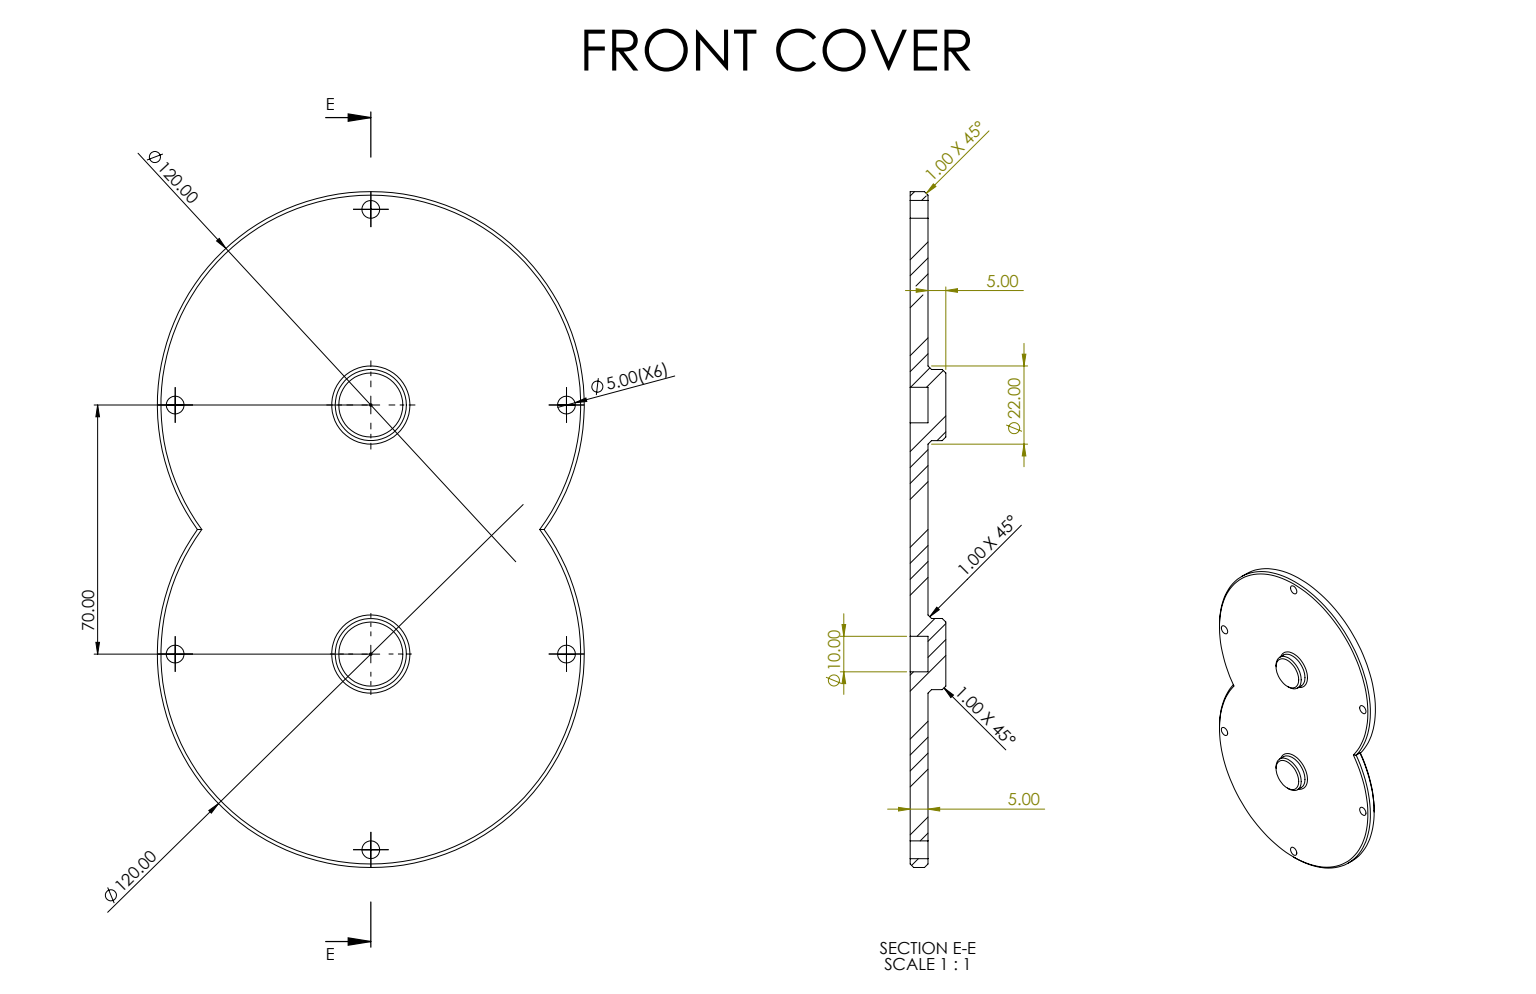
ISO-10303-21;
HEADER;
FILE_DESCRIPTION (('STEP AP214'),
    '1' );
FILE_NAME ('FRONT COVER.step',
    '2026-10-24T00:51:42',
    ( '' ),
    ( '' ),
    'SwSTEP 2.0',
    'SolidWorks 2025',
    '' );
FILE_SCHEMA (( 'AUTOMOTIVE_DESIGN' ));
ENDSEC;

DATA;
#13=ORIENTED_EDGE ( 'NONE', *, *, #8232, .T. ) ;
#20=CIRCLE ( 'NONE', #20518, 59.99999999999703704 ) ;
#28=DIRECTION ( 'NONE',  ( 0.000000000000000000, 1.000000000000000000, 0.000000000000000000 ) ) ;
#51=DIRECTION ( 'NONE',  ( 0.000000000000000000, 0.000000000000000000, -1.000000000000000000 ) ) ;
#74=VECTOR ( 'NONE', #6196, 1000.000000000000114 ) ;
#113=DIRECTION ( 'NONE',  ( 0.000000000000000000, 0.000000000000000000, 1.000000000000000000 ) ) ;
#181=DIRECTION ( 'NONE',  ( 8.659560562354903276E-17, -0.7071067811865500152, 0.7071067811865451302 ) ) ;
#196=EDGE_CURVE ( 'NONE', #9340, #20230, #6736, .T. ) ;
#205=CYLINDRICAL_SURFACE ( 'NONE', #8297, 59.99999999999700862 ) ;
#210=CARTESIAN_POINT ( 'NONE',  ( 35.00000000000001421, 5.000000000000000000, 1.540743955509788682E-30 ) ) ;
#215=DIRECTION ( 'NONE',  ( 0.000000000000000000, 1.000000000000000000, 0.000000000000000000 ) ) ;
#224=ORIENTED_EDGE ( 'NONE', *, *, #266, .F. ) ;
#225=CARTESIAN_POINT ( 'NONE',  ( 35.00000000000001421, 5.000000000000000000, 1.540743955509788682E-30 ) ) ;
#227=CARTESIAN_POINT ( 'NONE',  ( -34.99999999999999289, 0.000000000000000000, -3.012171160963566127E-14 ) ) ;
#265=CYLINDRICAL_SURFACE ( 'NONE', #18235, 10.00000000000000000 ) ;
#266=EDGE_CURVE ( 'NONE', #2332, #7531, #8895, .T. ) ;
#277=ADVANCED_FACE ( 'NONE', ( #12548, #8677, #5469, #19561, #10835, #1813, #15871, #8796, #9131 ), #15657, .T. ) ;
#288=DIRECTION ( 'NONE',  ( 0.000000000000000000, 0.000000000000000000, -1.000000000000000000 ) ) ;
#300=CARTESIAN_POINT ( 'NONE',  ( -34.99999999999999289, -5.000000000000000000, -54.99999999999705125 ) ) ;
#347=DIRECTION ( 'NONE',  ( 0.000000000000000000, 1.000000000000000000, 0.000000000000000000 ) ) ;
#353=VERTEX_POINT ( 'NONE', #21620 ) ;
#368=EDGE_LOOP ( 'NONE', ( #6095, #15311 ) ) ;
#460=ORIENTED_EDGE ( 'NONE', *, *, #7404, .T. ) ;
#474=CONICAL_SURFACE ( 'NONE', #18047, 58.99999999999701572, 0.7853981633974447263 ) ;
#508=ORIENTED_EDGE ( 'NONE', *, *, #14045, .T. ) ;
#516=CARTESIAN_POINT ( 'NONE',  ( -34.99999999999999289, 0.000000000000000000, -3.012171160963566127E-14 ) ) ;
#534=ORIENTED_EDGE ( 'NONE', *, *, #12604, .F. ) ;
#595=CIRCLE ( 'NONE', #3894, 10.00000000000000000 ) ;
#616=FACE_OUTER_BOUND ( 'NONE', #2436, .T. ) ;
#624=AXIS2_PLACEMENT_3D ( 'NONE', #14990, #8139, #11902 ) ;
#635=VECTOR ( 'NONE', #1063, 1000.000000000000114 ) ;
#664=DIRECTION ( 'NONE',  ( 0.000000000000000000, 1.000000000000000000, 0.000000000000000000 ) ) ;
#672=CARTESIAN_POINT ( 'NONE',  ( 34.99999999999999289, 0.000000000000000000, -57.49999999999705835 ) ) ;
#699=LINE ( 'NONE', #7682, #18205 ) ;
#717=ORIENTED_EDGE ( 'NONE', *, *, #8304, .F. ) ;
#734=ORIENTED_EDGE ( 'NONE', *, *, #2868, .F. ) ;
#762=DIRECTION ( 'NONE',  ( 0.000000000000000000, 1.000000000000000000, 0.000000000000000000 ) ) ;
#805=ADVANCED_FACE ( 'NONE', ( #10988 ), #3257, .T. ) ;
#830=ORIENTED_EDGE ( 'NONE', *, *, #3767, .F. ) ;
#840=CARTESIAN_POINT ( 'NONE',  ( -0.2854126906103648387, -4.332981472378772736, -48.52899265465751455 ) ) ;
#864=CARTESIAN_POINT ( 'NONE',  ( -89.99999999999701572, -5.000000000000000000, -3.012171160963566127E-14 ) ) ;
#904=EDGE_CURVE ( 'NONE', #353, #12856, #6012, .T. ) ;
#944=CARTESIAN_POINT ( 'NONE',  ( 34.99999999999999289, -5.000000000000000000, -54.99999999999705835 ) ) ;
#950=VERTEX_POINT ( 'NONE', #9985 ) ;
#959=ORIENTED_EDGE ( 'NONE', *, *, #1342, .F. ) ;
#960=UNCERTAINTY_MEASURE_WITH_UNIT (LENGTH_MEASURE( 1.000000000000000082E-05 ), #19624, 'distance_accuracy_value', 'NONE');
#982=EDGE_LOOP ( 'NONE', ( #22438, #1446 ) ) ;
#993=ORIENTED_EDGE ( 'NONE', *, *, #18740, .F. ) ;
#997=CARTESIAN_POINT ( 'NONE',  ( -34.99999999999999289, 0.000000000000000000, -58.99999999999701572 ) ) ;
#1011=CARTESIAN_POINT ( 'NONE',  ( 35.00000000000001421, -5.000000000000000000, 1.540743955509788682E-30 ) ) ;
#1015=ORIENTED_EDGE ( 'NONE', *, *, #2081, .T. ) ;
#1027=DIRECTION ( 'NONE',  ( 0.000000000000000000, -1.000000000000000000, 0.000000000000000000 ) ) ;
#1035=DIRECTION ( 'NONE',  ( 5.292376706370188309E-15, 0.000000000000000000, 1.000000000000000000 ) ) ;
#1039=FACE_OUTER_BOUND ( 'NONE', #8515, .T. ) ;
#1063=DIRECTION ( 'NONE',  ( 0.000000000000000000, 0.7071067811865549002, 0.7071067811865402453 ) ) ;
#1065=ORIENTED_EDGE ( 'NONE', *, *, #16608, .T. ) ;
#1105=AXIS2_PLACEMENT_3D ( 'NONE', #8719, #1616, #8487 ) ;
#1153=DIRECTION ( 'NONE',  ( 0.000000000000000000, 1.000000000000000000, 0.000000000000000000 ) ) ;
#1160=ADVANCED_FACE ( 'NONE', ( #14426 ), #18742, .T. ) ;
#1180=DIRECTION ( 'NONE',  ( 0.000000000000000000, 1.000000000000000000, 0.000000000000000000 ) ) ;
#1201=ADVANCED_FACE ( 'NONE', ( #7344 ), #11115, .F. ) ;
#1208=ORIENTED_EDGE ( 'NONE', *, *, #15769, .F. ) ;
#1214=VECTOR ( 'NONE', #15855, 1000.000000000000000 ) ;
#1223=CARTESIAN_POINT ( 'NONE',  ( -0.5687583343899673682, -4.666323447581315342, 48.32169744526331812 ) ) ;
#1247=CARTESIAN_POINT ( 'NONE',  ( 89.99999999999701572, 0.000000000000000000, -2.500000000000060840 ) ) ;
#1252=ORIENTED_EDGE ( 'NONE', *, *, #21699, .F. ) ;
#1259=ORIENTED_EDGE ( 'NONE', *, *, #15717, .F. ) ;
#1264=EDGE_CURVE ( 'NONE', #4080, #2931, #22007, .T. ) ;
#1272=LINE ( 'NONE', #4387, #9795 ) ;
#1273=CARTESIAN_POINT ( 'NONE',  ( -34.99999999999999289, -1.000000000000028644, -3.012171160963566127E-14 ) ) ;
#1277=VERTEX_POINT ( 'NONE', #9857 ) ;
#1313=VECTOR ( 'NONE', #19787, 1000.000000000000000 ) ;
#1321=LINE ( 'NONE', #11407, #12067 ) ;
#1333=EDGE_CURVE ( 'NONE', #7707, #18834, #16846, .T. ) ;
#1342=EDGE_CURVE ( 'NONE', #6332, #11390, #20202, .T. ) ;
#1345=ORIENTED_EDGE ( 'NONE', *, *, #1728, .F. ) ;
#1351=CARTESIAN_POINT ( 'NONE',  ( -34.99999999999999289, 0.000000000000000000, -54.99999999999705125 ) ) ;
#1357=ORIENTED_EDGE ( 'NONE', *, *, #7511, .T. ) ;
#1360=ORIENTED_EDGE ( 'NONE', *, *, #8232, .F. ) ;
#1361=DIRECTION ( 'NONE',  ( 0.000000000000000000, 0.000000000000000000, 1.000000000000000000 ) ) ;
#1377=EDGE_CURVE ( 'NONE', #9166, #8764, #11774, .T. ) ;
#1381=AXIS2_PLACEMENT_3D ( 'NONE', #8599, #1617, #10533 ) ;
#1419=ORIENTED_EDGE ( 'NONE', *, *, #5332, .F. ) ;
#1421=ORIENTED_EDGE ( 'NONE', *, *, #8605, .F. ) ;
#1422=EDGE_CURVE ( 'NONE', #6590, #6061, #10662, .T. ) ;
#1424=DIRECTION ( 'NONE',  ( 0.000000000000000000, 0.000000000000000000, -1.000000000000000000 ) ) ;
#1446=ORIENTED_EDGE ( 'NONE', *, *, #8571, .T. ) ;
#1452=B_SPLINE_CURVE_WITH_KNOTS ( 'NONE', 3,
 ( #13805, #20822, #11366, #2671 ),
 .UNSPECIFIED., .F., .F.,
 ( 4, 4 ),
 ( 0.000000000000000000, 0.001590342073036659634 ),
 .UNSPECIFIED. ) ;
#1490=FACE_OUTER_BOUND ( 'NONE', #12539, .T. ) ;
#1500=VERTEX_POINT ( 'NONE', #10137 ) ;
#1504=DIRECTION ( 'NONE',  ( 0.000000000000000000, 1.000000000000000000, 0.000000000000000000 ) ) ;
#1519=ORIENTED_EDGE ( 'NONE', *, *, #4640, .F. ) ;
#1543=CARTESIAN_POINT ( 'NONE',  ( 35.00000000000002132, -5.000000000000000000, -59.99999999999703704 ) ) ;
#1559=CARTESIAN_POINT ( 'NONE',  ( -34.99999999999999289, -5.000000000000000000, -52.49999999999705125 ) ) ;
#1604=DIRECTION ( 'NONE',  ( 0.000000000000000000, 0.000000000000000000, 1.000000000000000000 ) ) ;
#1616=DIRECTION ( 'NONE',  ( 0.000000000000000000, 1.000000000000000000, 0.000000000000000000 ) ) ;
#1617=DIRECTION ( 'NONE',  ( 0.000000000000000000, -1.000000000000000000, 0.000000000000000000 ) ) ;
#1637=DIRECTION ( 'NONE',  ( 0.000000000000000000, 1.000000000000000000, 0.000000000000000000 ) ) ;
#1648=CARTESIAN_POINT ( 'NONE',  ( 0.000000000000000000, 0.000000000000000000, 0.000000000000000000 ) ) ;
#1660=DIRECTION ( 'NONE',  ( 0.000000000000000000, 0.000000000000000000, -1.000000000000000000 ) ) ;
#1671=ORIENTED_EDGE ( 'NONE', *, *, #14527, .T. ) ;
#1675=AXIS2_PLACEMENT_3D ( 'NONE', #11723, #4855, #15373 ) ;
#1685=ORIENTED_EDGE ( 'NONE', *, *, #19206, .T. ) ;
#1689=DIRECTION ( 'NONE',  ( 0.000000000000000000, 1.000000000000000000, 0.000000000000000000 ) ) ;
#1710=LINE ( 'NONE', #16802, #7044 ) ;
#1711=LINE ( 'NONE', #14047, #14166 ) ;
#1717=DIRECTION ( 'NONE',  ( 0.000000000000000000, 1.000000000000000000, 0.000000000000000000 ) ) ;
#1728=EDGE_CURVE ( 'NONE', #11390, #6332, #7045, .T. ) ;
#1733=FACE_OUTER_BOUND ( 'NONE', #6732, .T. ) ;
#1757=AXIS2_PLACEMENT_3D ( 'NONE', #9404, #14192, #10999 ) ;
#1767=VERTEX_POINT ( 'NONE', #11621 ) ;
#1778=VECTOR ( 'NONE', #2503, 1000.000000000000000 ) ;
#1791=AXIS2_PLACEMENT_3D ( 'NONE', #4033, #12375, #113 ) ;
#1813=FACE_BOUND ( 'NONE', #15683, .T. ) ;
#1839=EDGE_CURVE ( 'NONE', #3030, #17217, #20670, .T. ) ;
#1853=CARTESIAN_POINT ( 'NONE',  ( -34.99999999999999289, -5.000000000000000000, 4.999999999999969802 ) ) ;
#1867=AXIS2_PLACEMENT_3D ( 'NONE', #14446, #11021, #16064 ) ;
#1901=LINE ( 'NONE', #8880, #1214 ) ;
#1902=ADVANCED_FACE ( 'NONE', ( #11839 ), #12486, .T. ) ;
#1946=DIRECTION ( 'NONE',  ( 0.000000000000000000, 0.000000000000000000, 1.000000000000000000 ) ) ;
#1951=FACE_BOUND ( 'NONE', #22385, .T. ) ;
#1952=AXIS2_PLACEMENT_3D ( 'NONE', #9959, #4929, #22467 ) ;
#1967=AXIS2_PLACEMENT_3D ( 'NONE', #22562, #6856, #13822 ) ;
#1970=CIRCLE ( 'NONE', #3085, 4.999999999999997335 ) ;
#1987=EDGE_CURVE ( 'NONE', #9166, #6590, #21289, .T. ) ;
#2033=CARTESIAN_POINT ( 'NONE',  ( 34.99999999999999289, 0.000000000000000000, -54.99999999999705835 ) ) ;
#2036=CARTESIAN_POINT ( 'NONE',  ( 35.00000000000001421, 5.000000000000000000, 1.540743955509788682E-30 ) ) ;
#2064=DIRECTION ( 'NONE',  ( 0.000000000000000000, 1.000000000000000000, 0.000000000000000000 ) ) ;
#2074=ORIENTED_EDGE ( 'NONE', *, *, #1422, .T. ) ;
#2080=LINE ( 'NONE', #5746, #14555 ) ;
#2081=EDGE_CURVE ( 'NONE', #10039, #14190, #11408, .T. ) ;
#2085=ORIENTED_EDGE ( 'NONE', *, *, #12937, .F. ) ;
#2100=CARTESIAN_POINT ( 'NONE',  ( 35.00000000000001421, -5.000000000000000000, 4.999999999999997335 ) ) ;
#2102=ORIENTED_EDGE ( 'NONE', *, *, #14902, .T. ) ;
#2105=LINE ( 'NONE', #14117, #16305 ) ;
#2113=AXIS2_PLACEMENT_3D ( 'NONE', #6299, #2756, #13257 ) ;
#2123=ORIENTED_EDGE ( 'NONE', *, *, #4379, .T. ) ;
#2142=DIRECTION ( 'NONE',  ( 0.000000000000000000, 1.000000000000000000, 0.000000000000000000 ) ) ;
#2199=VERTEX_POINT ( 'NONE', #15694 ) ;
#2204=( NAMED_UNIT ( * ) PLANE_ANGLE_UNIT ( ) SI_UNIT ( $, .RADIAN. ) );
#2205=ORIENTED_EDGE ( 'NONE', *, *, #15691, .F. ) ;
#2234=ORIENTED_EDGE ( 'NONE', *, *, #20437, .T. ) ;
#2261=DIRECTION ( 'NONE',  ( 0.000000000000000000, 1.000000000000000000, 0.000000000000000000 ) ) ;
#2285=ORIENTED_EDGE ( 'NONE', *, *, #3044, .T. ) ;
#2310=EDGE_LOOP ( 'NONE', ( #20692, #6820, #17268, #1015, #21602, #6129 ) ) ;
#2332=VERTEX_POINT ( 'NONE', #12582 ) ;
#2341=ADVANCED_FACE ( 'NONE', ( #16259 ), #19718, .T. ) ;
#2357=DIRECTION ( 'NONE',  ( 0.000000000000000000, 0.000000000000000000, 1.000000000000000000 ) ) ;
#2392=CARTESIAN_POINT ( 'NONE',  ( -34.99999999999999289, -3.999999999999985345, -3.012171160963566127E-14 ) ) ;
#2393=CONICAL_SURFACE ( 'NONE', #10411, 59.99999999999700862, 0.7853981633974380649 ) ;
#2396=AXIS2_PLACEMENT_3D ( 'NONE', #17885, #21211, #7342 ) ;
#2419=AXIS2_PLACEMENT_3D ( 'NONE', #20940, #1689, #8221 ) ;
#2427=EDGE_CURVE ( 'NONE', #22344, #3030, #8546, .T. ) ;
#2436=EDGE_LOOP ( 'NONE', ( #20453, #6374, #6252, #19334 ) ) ;
#2458=CARTESIAN_POINT ( 'NONE',  ( -34.99999999999999289, 0.000000000000000000, -3.012171160963566127E-14 ) ) ;
#2460=ORIENTED_EDGE ( 'NONE', *, *, #10047, .T. ) ;
#2472=VERTEX_POINT ( 'NONE', #1559 ) ;
#2484=CYLINDRICAL_SURFACE ( 'NONE', #16671, 59.99999999999703704 ) ;
#2503=DIRECTION ( 'NONE',  ( -0.000000000000000000, -1.000000000000000000, -0.000000000000000000 ) ) ;
#2523=ORIENTED_EDGE ( 'NONE', *, *, #16926, .T. ) ;
#2529=DIRECTION ( 'NONE',  ( 0.000000000000000000, 0.000000000000000000, 1.000000000000000000 ) ) ;
#2548=PRODUCT ( 'FRONT COVER', 'FRONT COVER', '', ( #6769 ) ) ;
#2564=CARTESIAN_POINT ( 'NONE',  ( -34.99999999999999289, 0.000000000000000000, -57.49999999999705125 ) ) ;
#2596=EDGE_CURVE ( 'NONE', #14190, #8015, #20812, .T. ) ;
#2643=PLANE ( 'NONE',  #3678 ) ;
#2671=CARTESIAN_POINT ( 'NONE',  ( -2.783226368218592341E-14, 0.000000000000000000, 47.49736834814792985 ) ) ;
#2688=DIRECTION ( 'NONE',  ( 0.000000000000000000, 0.000000000000000000, 1.000000000000000000 ) ) ;
#2706=CIRCLE ( 'NONE', #22101, 11.00000000000003730 ) ;
#2710=DIRECTION ( 'NONE',  ( 0.000000000000000000, 1.000000000000000000, 0.000000000000000000 ) ) ;
#2726=LINE ( 'NONE', #17958, #7374 ) ;
#2746=AXIS2_PLACEMENT_3D ( 'NONE', #6857, #22684, #20946 ) ;
#2756=DIRECTION ( 'NONE',  ( -0.000000000000000000, -1.000000000000000000, -0.000000000000000000 ) ) ;
#2782=ORIENTED_EDGE ( 'NONE', *, *, #14527, .F. ) ;
#2783=FACE_OUTER_BOUND ( 'NONE', #16329, .T. ) ;
#2790=EDGE_LOOP ( 'NONE', ( #508, #9529 ) ) ;
#2830=ORIENTED_EDGE ( 'NONE', *, *, #10117, .T. ) ;
#2836=DIRECTION ( 'NONE',  ( -0.000000000000000000, 1.000000000000000000, -0.000000000000000000 ) ) ;
#2840=VERTEX_POINT ( 'NONE', #20675 ) ;
#2863=VECTOR ( 'NONE', #17832, 1000.000000000000114 ) ;
#2867=DIRECTION ( 'NONE',  ( 1.734723475976892686E-15, 0.000000000000000000, 1.000000000000000000 ) ) ;
#2868=EDGE_CURVE ( 'NONE', #12296, #7531, #10896, .T. ) ;
#2875=VERTEX_POINT ( 'NONE', #15498 ) ;
#2891=EDGE_LOOP ( 'NONE', ( #17547, #17921, #11604, #5644 ) ) ;
#2908=DIRECTION ( 'NONE',  ( 0.000000000000000000, 1.000000000000000000, 0.000000000000000000 ) ) ;
#2909=DIRECTION ( 'NONE',  ( 0.000000000000000000, 1.000000000000000000, 0.000000000000000000 ) ) ;
#2931=VERTEX_POINT ( 'NONE', #4163 ) ;
#2972=ORIENTED_EDGE ( 'NONE', *, *, #3652, .F. ) ;
#2990=CARTESIAN_POINT ( 'NONE',  ( -34.99999999999998579, -3.999999999999985345, -59.99999999999703704 ) ) ;
#2996=EDGE_LOOP ( 'NONE', ( #4896, #14681, #2460, #14741, #12315, #14007 ) ) ;
#3001=ORIENTED_EDGE ( 'NONE', *, *, #3202, .F. ) ;
#3009=DIRECTION ( 'NONE',  ( -0.000000000000000000, 1.000000000000000000, -0.000000000000000000 ) ) ;
#3014=CARTESIAN_POINT ( 'NONE',  ( -34.99999999999999289, 4.000000000000028422, -3.012171160963566127E-14 ) ) ;
#3030=VERTEX_POINT ( 'NONE', #12739 ) ;
#3044=EDGE_CURVE ( 'NONE', #4376, #13677, #16435, .T. ) ;
#3050=EDGE_LOOP ( 'NONE', ( #11360, #15711 ) ) ;
#3077=VERTEX_POINT ( 'NONE', #9876 ) ;
#3085=AXIS2_PLACEMENT_3D ( 'NONE', #4024, #9509, #21544 ) ;
#3097=ORIENTED_EDGE ( 'NONE', *, *, #1333, .F. ) ;
#3111=FACE_OUTER_BOUND ( 'NONE', #22167, .T. ) ;
#3131=DIRECTION ( 'NONE',  ( 0.000000000000000000, 0.000000000000000000, 1.000000000000000000 ) ) ;
#3142=ORIENTED_EDGE ( 'NONE', *, *, #8081, .T. ) ;
#3143=B_SPLINE_CURVE_WITH_KNOTS ( 'NONE', 3,
 ( #16538, #20211, #840, #21819 ),
 .UNSPECIFIED., .F., .F.,
 ( 4, 4 ),
 ( 0.000000000000000000, 0.001452302087772874839 ),
 .UNSPECIFIED. ) ;
#3148=EDGE_LOOP ( 'NONE', ( #12892, #6241 ) ) ;
#3164=ADVANCED_FACE ( 'NONE', ( #2783 ), #9475, .T. ) ;
#3187=ORIENTED_EDGE ( 'NONE', *, *, #12577, .F. ) ;
#3202=EDGE_CURVE ( 'NONE', #4584, #7707, #16799, .T. ) ;
#3206=AXIS2_PLACEMENT_3D ( 'NONE', #16063, #3935, #17905 ) ;
#3215=CIRCLE ( 'NONE', #2113, 11.00000000000003730 ) ;
#3219=EDGE_LOOP ( 'NONE', ( #15771, #11245, #13002, #1519 ) ) ;
#3244=EDGE_LOOP ( 'NONE', ( #15424, #19591 ) ) ;
#3257=CYLINDRICAL_SURFACE ( 'NONE', #3822, 10.00000000000000000 ) ;
#3280=CARTESIAN_POINT ( 'NONE',  ( 89.99999999999701572, 0.000000000000000000, -5.216535399428728743E-14 ) ) ;
#3331=CARTESIAN_POINT ( 'NONE',  ( -34.99999999999999289, -5.000000000000000000, -3.012171160963566127E-14 ) ) ;
#3332=ORIENTED_EDGE ( 'NONE', *, *, #6770, .F. ) ;
#3370=EDGE_LOOP ( 'NONE', ( #18621, #9458 ) ) ;
#3408=DIRECTION ( 'NONE',  ( 0.000000000000000000, 0.000000000000000000, 1.000000000000000000 ) ) ;
#3410=DIRECTION ( 'NONE',  ( 0.000000000000000000, 1.000000000000000000, 0.000000000000000000 ) ) ;
#3419=ADVANCED_FACE ( 'NONE', ( #10639, #10997, #21097, #21428, #1951, #12818, #7563, #10877, #5396 ), #19830, .F. ) ;
#3431=DIRECTION ( 'NONE',  ( 0.000000000000000000, 1.000000000000000000, 0.000000000000000000 ) ) ;
#3436=EDGE_CURVE ( 'NONE', #2840, #5633, #16413, .T. ) ;
#3441=AXIS2_PLACEMENT_3D ( 'NONE', #210, #7322, #9038 ) ;
#3444=VECTOR ( 'NONE', #1153, 1000.000000000000000 ) ;
#3454=SHAPE_DEFINITION_REPRESENTATION ( #16821, #13507 ) ;
#3460=DIRECTION ( 'NONE',  ( 0.000000000000000000, -1.000000000000000000, 0.000000000000000000 ) ) ;
#3496=VERTEX_POINT ( 'NONE', #14304 ) ;
#3524=ORIENTED_EDGE ( 'NONE', *, *, #4411, .F. ) ;
#3525=DIRECTION ( 'NONE',  ( 0.000000000000000000, 1.000000000000000000, -0.000000000000000000 ) ) ;
#3528=B_SPLINE_CURVE_WITH_KNOTS ( 'NONE', 3,
 ( #6847, #8220, #1223, #11762 ),
 .UNSPECIFIED., .F., .F.,
 ( 4, 4 ),
 ( 0.000000000000000000, 0.001452302087772880043 ),
 .UNSPECIFIED. ) ;
#3530=DIRECTION ( 'NONE',  ( 0.000000000000000000, 0.000000000000000000, 1.000000000000000000 ) ) ;
#3563=DIRECTION ( 'NONE',  ( 0.000000000000000000, 1.000000000000000000, 0.000000000000000000 ) ) ;
#3570=DIRECTION ( 'NONE',  ( 0.000000000000000000, 1.000000000000000000, 0.000000000000000000 ) ) ;
#3581=DIRECTION ( 'NONE',  ( 0.000000000000000000, 1.000000000000000000, 0.000000000000000000 ) ) ;
#3631=AXIS2_PLACEMENT_3D ( 'NONE', #16764, #9658, #8064 ) ;
#3652=EDGE_CURVE ( 'NONE', #11550, #1500, #6318, .T. ) ;
#3659=ORIENTED_EDGE ( 'NONE', *, *, #266, .T. ) ;
#3664=FACE_OUTER_BOUND ( 'NONE', #2790, .T. ) ;
#3678=AXIS2_PLACEMENT_3D ( 'NONE', #19935, #8024, #14982 ) ;
#3711=DIRECTION ( 'NONE',  ( 0.000000000000000000, 0.000000000000000000, 1.000000000000000000 ) ) ;
#3730=CARTESIAN_POINT ( 'NONE',  ( -34.99999999999999289, -3.999999999999985345, -3.012171160963566127E-14 ) ) ;
#3742=CARTESIAN_POINT ( 'NONE',  ( -34.99999999999997868, 0.000000000000000000, 54.99999999999698730 ) ) ;
#3758=EDGE_LOOP ( 'NONE', ( #16747, #22171, #10337, #18642 ) ) ;
#3767=EDGE_CURVE ( 'NONE', #21906, #4376, #1710, .T. ) ;
#3790=DIRECTION ( 'NONE',  ( 0.000000000000000000, 0.000000000000000000, 1.000000000000000000 ) ) ;
#3813=ORIENTED_EDGE ( 'NONE', *, *, #19503, .T. ) ;
#3815=EDGE_LOOP ( 'NONE', ( #2074, #13522, #4848, #12384 ) ) ;
#3822=AXIS2_PLACEMENT_3D ( 'NONE', #16250, #17976, #6919 ) ;
#3849=DIRECTION ( 'NONE',  ( 0.000000000000000000, 0.000000000000000000, 1.000000000000000000 ) ) ;
#3894=AXIS2_PLACEMENT_3D ( 'NONE', #11883, #13478, #13700 ) ;
#3907=CARTESIAN_POINT ( 'NONE',  ( -34.99999999999999289, -5.000000000000000000, -3.012171160963566127E-14 ) ) ;
#3913=FACE_OUTER_BOUND ( 'NONE', #19433, .T. ) ;
#3916=DIRECTION ( 'NONE',  ( 0.000000000000000000, -1.000000000000000000, 0.000000000000000000 ) ) ;
#3922=ORIENTED_EDGE ( 'NONE', *, *, #4411, .T. ) ;
#3930=VERTEX_POINT ( 'NONE', #19360 ) ;
#3932=EDGE_CURVE ( 'NONE', #20230, #4376, #10098, .T. ) ;
#3935=DIRECTION ( 'NONE',  ( 0.000000000000000000, 1.000000000000000000, 0.000000000000000000 ) ) ;
#3944=ADVANCED_FACE ( 'NONE', ( #3664 ), #10615, .F. ) ;
#3963=AXIS2_PLACEMENT_3D ( 'NONE', #9358, #2142, #12886 ) ;
#3976=AXIS2_PLACEMENT_3D ( 'NONE', #8325, #2836, #6606 ) ;
#3982=AXIS2_PLACEMENT_3D ( 'NONE', #19031, #18371, #2688 ) ;
#3993=ORIENTED_EDGE ( 'NONE', *, *, #17293, .T. ) ;
#3996=AXIS2_PLACEMENT_3D ( 'NONE', #4739, #4618, #18250 ) ;
#4011=DIRECTION ( 'NONE',  ( -0.000000000000000000, 1.000000000000000000, -0.000000000000000000 ) ) ;
#4024=CARTESIAN_POINT ( 'NONE',  ( 35.00000000000001421, -5.000000000000000000, 1.540743955509788682E-30 ) ) ;
#4033=CARTESIAN_POINT ( 'NONE',  ( -34.99999999999999289, 4.000000000000028422, -3.012171160963566127E-14 ) ) ;
#4057=DIRECTION ( 'NONE',  ( 0.000000000000000000, 0.000000000000000000, 1.000000000000000000 ) ) ;
#4061=EDGE_LOOP ( 'NONE', ( #18011, #5121, #2523, #959 ) ) ;
#4063=CARTESIAN_POINT ( 'NONE',  ( -89.99999999999701572, 0.000000000000000000, 2.499999999999978684 ) ) ;
#4080=VERTEX_POINT ( 'NONE', #10264 ) ;
#4085=DIRECTION ( 'NONE',  ( 0.000000000000000000, 1.000000000000000000, 0.000000000000000000 ) ) ;
#4089=DIRECTION ( 'NONE',  ( -0.000000000000000000, -1.000000000000000000, -0.000000000000000000 ) ) ;
#4102=FACE_OUTER_BOUND ( 'NONE', #4209, .T. ) ;
#4132=DIRECTION ( 'NONE',  ( 0.000000000000000000, -0.000000000000000000, 1.000000000000000000 ) ) ;
#4137=CARTESIAN_POINT ( 'NONE',  ( -34.99999999999999289, 0.000000000000000000, -3.012171160963566127E-14 ) ) ;
#4153=ORIENTED_EDGE ( 'NONE', *, *, #15425, .T. ) ;
#4163=CARTESIAN_POINT ( 'NONE',  ( -34.99999999999999289, 0.000000000000000000, -11.00000000000006750 ) ) ;
#4201=CARTESIAN_POINT ( 'NONE',  ( 35.00000000000001421, -5.000000000000000000, 1.540743955509788682E-30 ) ) ;
#4209=EDGE_LOOP ( 'NONE', ( #11237, #6980, #15911, #7527 ) ) ;
#4211=CARTESIAN_POINT ( 'NONE',  ( 35.00000000000002132, -5.000000000000000000, -59.99999999999703704 ) ) ;
#4218=DIRECTION ( 'NONE',  ( 0.000000000000000000, 0.000000000000000000, 1.000000000000000000 ) ) ;
#4225=CARTESIAN_POINT ( 'NONE',  ( -34.99999999999999289, -5.000000000000000000, -54.99999999999705125 ) ) ;
#4235=AXIS2_PLACEMENT_3D ( 'NONE', #7172, #21047, #9126 ) ;
#4243=VECTOR ( 'NONE', #17120, 1000.000000000000000 ) ;
#4244=FACE_OUTER_BOUND ( 'NONE', #3050, .T. ) ;
#4250=DIRECTION ( 'NONE',  ( -0.000000000000000000, -1.000000000000000000, -0.000000000000000000 ) ) ;
#4254=CARTESIAN_POINT ( 'NONE',  ( 35.00000000000001421, 0.000000000000000000, 1.540743955509788682E-30 ) ) ;
#4257=DIRECTION ( 'NONE',  ( 0.000000000000000000, 0.000000000000000000, -1.000000000000000000 ) ) ;
#4311=ORIENTED_EDGE ( 'NONE', *, *, #5518, .F. ) ;
#4316=AXIS2_PLACEMENT_3D ( 'NONE', #18352, #3009, #13069 ) ;
#4322=CIRCLE ( 'NONE', #22253, 2.500000000000002220 ) ;
#4333=LINE ( 'NONE', #997, #6879 ) ;
#4341=DIRECTION ( 'NONE',  ( 0.000000000000000000, 0.000000000000000000, 1.000000000000000000 ) ) ;
#4344=VERTEX_POINT ( 'NONE', #12840 ) ;
#4358=AXIS2_PLACEMENT_3D ( 'NONE', #18098, #347, #4132 ) ;
#4365=CARTESIAN_POINT ( 'NONE',  ( 35.00000000000001421, -1.000000000000028644, 1.540743955509788682E-30 ) ) ;
#4376=VERTEX_POINT ( 'NONE', #19627 ) ;
#4379=EDGE_CURVE ( 'NONE', #13224, #13528, #22248, .T. ) ;
#4383=AXIS2_PLACEMENT_3D ( 'NONE', #15739, #12089, #51 ) ;
#4387=CARTESIAN_POINT ( 'NONE',  ( -34.99999999999998579, -3.999999999999985345, -59.99999999999703704 ) ) ;
#4411=EDGE_CURVE ( 'NONE', #13828, #11150, #1272, .T. ) ;
#4429=DIRECTION ( 'NONE',  ( 0.000000000000000000, 0.000000000000000000, 1.000000000000000000 ) ) ;
#4444=AXIS2_PLACEMENT_3D ( 'NONE', #1273, #6553, #13957 ) ;
#4445=DIRECTION ( 'NONE',  ( 0.000000000000000000, 0.000000000000000000, 1.000000000000000000 ) ) ;
#4458=CYLINDRICAL_SURFACE ( 'NONE', #14761, 59.99999999999703704 ) ;
#4539=AXIS2_PLACEMENT_3D ( 'NONE', #8996, #21607, #288 ) ;
#4543=DIRECTION ( 'NONE',  ( 0.000000000000000000, 1.000000000000000000, 0.000000000000000000 ) ) ;
#4558=DIRECTION ( 'NONE',  ( 0.000000000000000000, 0.000000000000000000, 1.000000000000000000 ) ) ;
#4584=VERTEX_POINT ( 'NONE', #17075 ) ;
#4606=AXIS2_PLACEMENT_3D ( 'NONE', #17348, #8424, #15393 ) ;
#4618=DIRECTION ( 'NONE',  ( 0.000000000000000000, -1.000000000000000000, 0.000000000000000000 ) ) ;
#4619=CARTESIAN_POINT ( 'NONE',  ( 35.00000000000001421, 5.000000000000000000, 9.000000000000035527 ) ) ;
#4640=EDGE_CURVE ( 'NONE', #15853, #12856, #2726, .T. ) ;
#4681=CYLINDRICAL_SURFACE ( 'NONE', #11906, 4.999999999999997335 ) ;
#4682=ADVANCED_FACE ( 'NONE', ( #6273 ), #16811, .T. ) ;
#4689=DIRECTION ( 'NONE',  ( 0.000000000000000000, 1.000000000000000000, 0.000000000000000000 ) ) ;
#4715=CARTESIAN_POINT ( 'NONE',  ( -34.99999999999999289, 0.000000000000000000, -52.49999999999705125 ) ) ;
#4729=ORIENTED_EDGE ( 'NONE', *, *, #3652, .T. ) ;
#4739=CARTESIAN_POINT ( 'NONE',  ( -34.99999999999999289, 5.000000000000000000, -3.012171160963566127E-14 ) ) ;
#4781=CIRCLE ( 'NONE', #7695, 5.000000000000000000 ) ;
#4786=DIRECTION ( 'NONE',  ( 0.000000000000000000, 1.000000000000000000, 0.000000000000000000 ) ) ;
#4789=DIRECTION ( 'NONE',  ( 0.000000000000000000, 1.000000000000000000, 0.000000000000000000 ) ) ;
#4809=CARTESIAN_POINT ( 'NONE',  ( -34.99999999999999289, 0.000000000000000000, -3.012171160963566127E-14 ) ) ;
#4829=EDGE_CURVE ( 'NONE', #11055, #19583, #22454, .T. ) ;
#4834=CYLINDRICAL_SURFACE ( 'NONE', #1105, 2.500000000000002220 ) ;
#4848=ORIENTED_EDGE ( 'NONE', *, *, #8479, .T. ) ;
#4855=DIRECTION ( 'NONE',  ( -0.000000000000000000, -1.000000000000000000, -0.000000000000000000 ) ) ;
#4876=CARTESIAN_POINT ( 'NONE',  ( -34.99999999999999289, -5.000000000000000000, 59.99999999999698019 ) ) ;
#4887=ORIENTED_EDGE ( 'NONE', *, *, #11836, .F. ) ;
#4896=ORIENTED_EDGE ( 'NONE', *, *, #1987, .F. ) ;
#4929=DIRECTION ( 'NONE',  ( 0.000000000000000000, -1.000000000000000000, 0.000000000000000000 ) ) ;
#4935=CIRCLE ( 'NONE', #2746, 2.500000000000002220 ) ;
#4949=DIRECTION ( 'NONE',  ( 0.000000000000000000, 1.000000000000000000, 0.000000000000000000 ) ) ;
#4972=VERTEX_POINT ( 'NONE', #7972 ) ;
#4981=CARTESIAN_POINT ( 'NONE',  ( 89.99999999999701572, 0.000000000000000000, 2.499999999999956479 ) ) ;
#4987=ADVANCED_BREP_SHAPE_REPRESENTATION ( '', ( #10654, #18273 ), #22681 ) ;
#5004=VERTEX_POINT ( 'NONE', #4981 ) ;
#5020=EDGE_LOOP ( 'NONE', ( #15013, #11391 ) ) ;
#5038=CIRCLE ( 'NONE', #14531, 10.00000000000000000 ) ;
#5056=CARTESIAN_POINT ( 'NONE',  ( -34.99999999999999289, 5.000000000000000000, 9.000000000000007105 ) ) ;
#5105=ORIENTED_EDGE ( 'NONE', *, *, #10161, .T. ) ;
#5108=ORIENTED_EDGE ( 'NONE', *, *, #1839, .F. ) ;
#5110=FACE_OUTER_BOUND ( 'NONE', #2891, .T. ) ;
#5121=ORIENTED_EDGE ( 'NONE', *, *, #6388, .F. ) ;
#5140=CIRCLE ( 'NONE', #19411, 2.500000000000002220 ) ;
#5156=FACE_OUTER_BOUND ( 'NONE', #9966, .T. ) ;
#5169=CARTESIAN_POINT ( 'NONE',  ( 7.943521403985130338E-15, 0.000000000000000000, -47.49736834814795827 ) ) ;
#5178=CARTESIAN_POINT ( 'NONE',  ( 89.99999999999701572, 0.000000000000000000, -5.216535399428728743E-14 ) ) ;
#5244=CARTESIAN_POINT ( 'NONE',  ( 1.387778780781445676E-14, -5.000000000000000000, -48.73397172404115452 ) ) ;
#5246=DIRECTION ( 'NONE',  ( 0.000000000000000000, -1.000000000000000000, 0.000000000000000000 ) ) ;
#5275=EDGE_CURVE ( 'NONE', #11150, #10311, #18947, .T. ) ;
#5299=DIRECTION ( 'NONE',  ( 0.000000000000000000, 1.000000000000000000, 0.000000000000000000 ) ) ;
#5305=CARTESIAN_POINT ( 'NONE',  ( -34.99999999999999289, -3.999999999999985345, -3.012171160963566127E-14 ) ) ;
#5309=ORIENTED_EDGE ( 'NONE', *, *, #12414, .F. ) ;
#5332=EDGE_CURVE ( 'NONE', #8764, #10311, #11483, .T. ) ;
#5361=EDGE_CURVE ( 'NONE', #19717, #22344, #7818, .T. ) ;
#5388=DIRECTION ( 'NONE',  ( 0.000000000000000000, 0.000000000000000000, -1.000000000000000000 ) ) ;
#5391=FACE_OUTER_BOUND ( 'NONE', #16847, .T. ) ;
#5393=CARTESIAN_POINT ( 'NONE',  ( 35.00000000000001421, -5.000000000000000000, 1.540743955509788682E-30 ) ) ;
#5394=CONICAL_SURFACE ( 'NONE', #20045, 10.00000000000000000, 0.7853981633974447263 ) ;
#5396=FACE_OUTER_BOUND ( 'NONE', #2996, .T. ) ;
#5400=LINE ( 'NONE', #1853, #10060 ) ;
#5437=AXIS2_PLACEMENT_3D ( 'NONE', #11057, #4089, #16675 ) ;
#5469=FACE_BOUND ( 'NONE', #17372, .T. ) ;
#5474=CIRCLE ( 'NONE', #16448, 2.500000000000002220 ) ;
#5518=EDGE_CURVE ( 'NONE', #4344, #353, #17541, .T. ) ;
#5523=ORIENTED_EDGE ( 'NONE', *, *, #11051, .F. ) ;
#5532=DIRECTION ( 'NONE',  ( 0.000000000000000000, 1.000000000000000000, 0.000000000000000000 ) ) ;
#5547=EDGE_CURVE ( 'NONE', #4344, #15853, #13821, .T. ) ;
#5549=AXIS2_PLACEMENT_3D ( 'NONE', #21339, #16287, #14216 ) ;
#5574=VERTEX_POINT ( 'NONE', #1247 ) ;
#5590=DIRECTION ( 'NONE',  ( 0.000000000000000000, 0.000000000000000000, 1.000000000000000000 ) ) ;
#5633=VERTEX_POINT ( 'NONE', #9853 ) ;
#5644=ORIENTED_EDGE ( 'NONE', *, *, #5957, .F. ) ;
#5700=DIRECTION ( 'NONE',  ( 0.000000000000000000, 1.000000000000000000, -0.000000000000000000 ) ) ;
#5701=CYLINDRICAL_SURFACE ( 'NONE', #12448, 10.00000000000000000 ) ;
#5702=CARTESIAN_POINT ( 'NONE',  ( 35.00000000000001421, -1.000000000000028644, 1.540743955509788682E-30 ) ) ;
#5746=CARTESIAN_POINT ( 'NONE',  ( 35.00000000000001421, 5.000000000000000000, -10.00000000000000000 ) ) ;
#5804=AXIS2_PLACEMENT_3D ( 'NONE', #8668, #3525, #12106 ) ;
#5832=EDGE_CURVE ( 'NONE', #1767, #13224, #1711, .T. ) ;
#5839=CARTESIAN_POINT ( 'NONE',  ( -34.99999999999999289, 0.000000000000000000, -3.012171160963566127E-14 ) ) ;
#5890=CARTESIAN_POINT ( 'NONE',  ( 35.00000000000000000, -5.000000000000000000, 54.99999999999698019 ) ) ;
#5911=ORIENTED_EDGE ( 'NONE', *, *, #16926, .F. ) ;
#5913=LINE ( 'NONE', #12879, #7242 ) ;
#5915=DIRECTION ( 'NONE',  ( 0.000000000000000000, 1.000000000000000000, 0.000000000000000000 ) ) ;
#5926=CARTESIAN_POINT ( 'NONE',  ( -3.469446951953614189E-14, -3.999999999999985345, 48.73397172404114031 ) ) ;
#5932=CARTESIAN_POINT ( 'NONE',  ( -34.99999999999999289, -3.999999999999985345, -3.012171160963566127E-14 ) ) ;
#5957=EDGE_CURVE ( 'NONE', #2840, #4080, #14512, .T. ) ;
#6012=CIRCLE ( 'NONE', #15868, 2.500000000000002220 ) ;
#6022=CARTESIAN_POINT ( 'NONE',  ( -34.99999999999999289, 5.000000000000000000, -3.012171160963566127E-14 ) ) ;
#6061=VERTEX_POINT ( 'NONE', #1543 ) ;
#6089=CIRCLE ( 'NONE', #13752, 2.500000000000002220 ) ;
#6095=ORIENTED_EDGE ( 'NONE', *, *, #11836, .T. ) ;
#6100=CYLINDRICAL_SURFACE ( 'NONE', #11363, 2.500000000000002220 ) ;
#6119=CIRCLE ( 'NONE', #17763, 59.99999999999700862 ) ;
#6129=ORIENTED_EDGE ( 'NONE', *, *, #15717, .T. ) ;
#6141=ORIENTED_EDGE ( 'NONE', *, *, #1987, .T. ) ;
#6149=CARTESIAN_POINT ( 'NONE',  ( -34.99999999999999289, 1.000000000000044187, 9.999999999999971578 ) ) ;
#6162=DIRECTION ( 'NONE',  ( 0.000000000000000000, 1.000000000000000000, 0.000000000000000000 ) ) ;
#6169=FACE_OUTER_BOUND ( 'NONE', #4061, .T. ) ;
#6175=FACE_OUTER_BOUND ( 'NONE', #22032, .T. ) ;
#6179=CARTESIAN_POINT ( 'NONE',  ( -34.99999999999999289, 0.000000000000000000, -58.99999999999702993 ) ) ;
#6184=ADVANCED_FACE ( 'NONE', ( #5110 ), #265, .T. ) ;
#6196=DIRECTION ( 'NONE',  ( 0.000000000000000000, -0.7071067811865500152, -0.7071067811865451302 ) ) ;
#6200=CYLINDRICAL_SURFACE ( 'NONE', #19551, 10.00000000000000000 ) ;
#6202=ORIENTED_EDGE ( 'NONE', *, *, #17180, .T. ) ;
#6241=ORIENTED_EDGE ( 'NONE', *, *, #8304, .T. ) ;
#6252=ORIENTED_EDGE ( 'NONE', *, *, #22220, .F. ) ;
#6273=FACE_OUTER_BOUND ( 'NONE', #6832, .T. ) ;
#6297=DIRECTION ( 'NONE',  ( 0.000000000000000000, 1.000000000000000000, 0.000000000000000000 ) ) ;
#6299=CARTESIAN_POINT ( 'NONE',  ( -34.99999999999999289, 0.000000000000000000, -3.012171160963566127E-14 ) ) ;
#6318=CIRCLE ( 'NONE', #19136, 2.500000000000002220 ) ;
#6326=ORIENTED_EDGE ( 'NONE', *, *, #5832, .T. ) ;
#6332=VERTEX_POINT ( 'NONE', #12854 ) ;
#6335=ORIENTED_EDGE ( 'NONE', *, *, #4640, .T. ) ;
#6342=ADVANCED_FACE ( 'NONE', ( #11606 ), #9887, .T. ) ;
#6374=ORIENTED_EDGE ( 'NONE', *, *, #19658, .F. ) ;
#6388=EDGE_CURVE ( 'NONE', #10638, #9680, #1970, .T. ) ;
#6398=FACE_OUTER_BOUND ( 'NONE', #16860, .T. ) ;
#6402=CLOSED_SHELL ( 'NONE', ( #11558, #15977, #21072, #17552, #10476, #3164, #18971, #1160, #7877, #11153, #8622, #6184, #18030, #15032, #8107, #18639, #7981, #8561, #12450, #1201, #21163, #4682, #15367, #6342, #11464, #17295, #3419, #277, #20808, #14905, #17848, #17728, #14298, #21900, #7231, #8117, #3944, #805, #17868, #8429, #10529, #8480, #10844, #18939, #1902, #9631, #14345, #2341, #19798 ) ) ;
#6404=CIRCLE ( 'NONE', #7120, 5.000000000000000000 ) ;
#6407=ORIENTED_EDGE ( 'NONE', *, *, #5547, .T. ) ;
#6408=CYLINDRICAL_SURFACE ( 'NONE', #15744, 2.500000000000002220 ) ;
#6419=DIRECTION ( 'NONE',  ( 0.000000000000000000, 1.000000000000000000, 0.000000000000000000 ) ) ;
#6457=ORIENTED_EDGE ( 'NONE', *, *, #9839, .T. ) ;
#6488=ORIENTED_EDGE ( 'NONE', *, *, #10845, .F. ) ;
#6516=ORIENTED_EDGE ( 'NONE', *, *, #8390, .T. ) ;
#6544=AXIS2_PLACEMENT_3D ( 'NONE', #944, #16868, #8159 ) ;
#6547=ORIENTED_EDGE ( 'NONE', *, *, #22476, .T. ) ;
#6553=DIRECTION ( 'NONE',  ( 0.000000000000000000, -1.000000000000000000, 0.000000000000000000 ) ) ;
#6557=LINE ( 'NONE', #18811, #13454 ) ;
#6590=VERTEX_POINT ( 'NONE', #20848 ) ;
#6595=LINE ( 'NONE', #4876, #4243 ) ;
#6606=DIRECTION ( 'NONE',  ( 0.000000000000000000, 0.000000000000000000, 1.000000000000000000 ) ) ;
#6626=CONICAL_SURFACE ( 'NONE', #1867, 58.99999999999701572, 0.7853981633974447263 ) ;
#6643=CARTESIAN_POINT ( 'NONE',  ( -2.783226368218592341E-14, 0.000000000000000000, 47.49736834814792985 ) ) ;
#6647=ORIENTED_EDGE ( 'NONE', *, *, #14045, .F. ) ;
#6671=CARTESIAN_POINT ( 'NONE',  ( -34.99999999999999289, -1.000000000000028644, 59.99999999999698019 ) ) ;
#6699=ORIENTED_EDGE ( 'NONE', *, *, #19535, .F. ) ;
#6727=CARTESIAN_POINT ( 'NONE',  ( -89.99999999999701572, -5.000000000000000000, -3.012171160963566127E-14 ) ) ;
#6732=EDGE_LOOP ( 'NONE', ( #13549, #6326, #2123, #1421 ) ) ;
#6736=LINE ( 'NONE', #10605, #21398 ) ;
#6739=AXIS2_PLACEMENT_3D ( 'NONE', #20066, #9523, #4257 ) ;
#6769=PRODUCT_CONTEXT ( 'NONE', #22052, 'mechanical' ) ;
#6770=EDGE_CURVE ( 'NONE', #6061, #14915, #11309, .T. ) ;
#6776=CARTESIAN_POINT ( 'NONE',  ( -34.99999999999999289, 1.000000000000044187, -3.012171160963566127E-14 ) ) ;
#6801=ORIENTED_EDGE ( 'NONE', *, *, #3044, .F. ) ;
#6820=ORIENTED_EDGE ( 'NONE', *, *, #15769, .T. ) ;
#6832=EDGE_LOOP ( 'NONE', ( #18506, #6999, #4153, #3142 ) ) ;
#6847=CARTESIAN_POINT ( 'NONE',  ( -3.469446951953614189E-14, -3.999999999999985345, 48.73397172404114031 ) ) ;
#6856=DIRECTION ( 'NONE',  ( 0.000000000000000000, 1.000000000000000000, 0.000000000000000000 ) ) ;
#6857=CARTESIAN_POINT ( 'NONE',  ( -34.99999999999999289, 0.000000000000000000, -54.99999999999705125 ) ) ;
#6879=VECTOR ( 'NONE', #11313, 1000.000000000000114 ) ;
#6910=EDGE_LOOP ( 'NONE', ( #22686, #3922, #18577, #2205 ) ) ;
#6911=DIRECTION ( 'NONE',  ( 0.000000000000000000, 0.000000000000000000, 1.000000000000000000 ) ) ;
#6919=DIRECTION ( 'NONE',  ( 0.000000000000000000, 0.000000000000000000, -1.000000000000000000 ) ) ;
#6938=ORIENTED_EDGE ( 'NONE', *, *, #8479, .F. ) ;
#6950=VERTEX_POINT ( 'NONE', #10029 ) ;
#6956=CARTESIAN_POINT ( 'NONE',  ( 35.00000000000001421, 5.000000000000000000, 10.00000000000000000 ) ) ;
#6968=DIRECTION ( 'NONE',  ( 0.000000000000000000, 1.000000000000000000, 0.000000000000000000 ) ) ;
#6980=ORIENTED_EDGE ( 'NONE', *, *, #10107, .F. ) ;
#6999=ORIENTED_EDGE ( 'NONE', *, *, #5275, .T. ) ;
#7018=DIRECTION ( 'NONE',  ( -0.000000000000000000, 1.000000000000000000, -0.000000000000000000 ) ) ;
#7040=DIRECTION ( 'NONE',  ( 0.000000000000000000, -0.7071067811865500152, -0.7071067811865450192 ) ) ;
#7043=FACE_OUTER_BOUND ( 'NONE', #6910, .T. ) ;
#7044=VECTOR ( 'NONE', #3431, 1000.000000000000000 ) ;
#7045=CIRCLE ( 'NONE', #13606, 4.999999999999997335 ) ;
#7049=EDGE_CURVE ( 'NONE', #7098, #3030, #15459, .T. ) ;
#7051=EDGE_LOOP ( 'NONE', ( #17936, #20219, #21551, #16822 ) ) ;
#7086=AXIS2_PLACEMENT_3D ( 'NONE', #3742, #14482, #19664 ) ;
#7098=VERTEX_POINT ( 'NONE', #7162 ) ;
#7099=VECTOR ( 'NONE', #11187, 1000.000000000000000 ) ;
#7111=CYLINDRICAL_SURFACE ( 'NONE', #2396, 59.99999999999700862 ) ;
#7120=AXIS2_PLACEMENT_3D ( 'NONE', #5839, #11207, #16485 ) ;
#7133=EDGE_CURVE ( 'NONE', #6590, #20230, #1901, .T. ) ;
#7157=AXIS2_PLACEMENT_3D ( 'NONE', #5305, #7018, #12278 ) ;
#7162=CARTESIAN_POINT ( 'NONE',  ( 35.00000000000001421, 1.000000000000044187, -10.00000000000000000 ) ) ;
#7172=CARTESIAN_POINT ( 'NONE',  ( -34.99999999999999289, 0.000000000000000000, -3.012171160963566127E-14 ) ) ;
#7173=CYLINDRICAL_SURFACE ( 'NONE', #20825, 2.500000000000002220 ) ;
#7181=DIRECTION ( 'NONE',  ( 0.000000000000000000, 0.000000000000000000, -1.000000000000000000 ) ) ;
#7218=DIRECTION ( 'NONE',  ( 0.000000000000000000, 0.000000000000000000, -1.000000000000000000 ) ) ;
#7231=ADVANCED_FACE ( 'NONE', ( #17820 ), #12987, .F. ) ;
#7242=VECTOR ( 'NONE', #19889, 1000.000000000000000 ) ;
#7249=ORIENTED_EDGE ( 'NONE', *, *, #10047, .F. ) ;
#7271=DIRECTION ( 'NONE',  ( 0.000000000000000000, 0.000000000000000000, 1.000000000000000000 ) ) ;
#7322=DIRECTION ( 'NONE',  ( 0.000000000000000000, 1.000000000000000000, 0.000000000000000000 ) ) ;
#7342=DIRECTION ( 'NONE',  ( 0.000000000000000000, 0.000000000000000000, 1.000000000000000000 ) ) ;
#7344=FACE_OUTER_BOUND ( 'NONE', #16998, .T. ) ;
#7351=CARTESIAN_POINT ( 'NONE',  ( -34.99999999999997868, 0.000000000000000000, 52.49999999999698730 ) ) ;
#7374=VECTOR ( 'NONE', #2261, 1000.000000000000000 ) ;
#7404=EDGE_CURVE ( 'NONE', #17217, #1277, #2706, .T. ) ;
#7416=AXIS2_PLACEMENT_3D ( 'NONE', #3730, #12196, #10682 ) ;
#7420=CARTESIAN_POINT ( 'NONE',  ( -34.99999999999999289, 5.000000000000000000, -10.00000000000003020 ) ) ;
#7472=( NAMED_UNIT ( * ) SI_UNIT ( $, .STERADIAN. ) SOLID_ANGLE_UNIT ( ) );
#7494=ORIENTED_EDGE ( 'NONE', *, *, #17293, .F. ) ;
#7511=EDGE_CURVE ( 'NONE', #16627, #10912, #21737, .T. ) ;
#7527=ORIENTED_EDGE ( 'NONE', *, *, #18287, .T. ) ;
#7531=VERTEX_POINT ( 'NONE', #12873 ) ;
#7542=AXIS2_PLACEMENT_3D ( 'NONE', #18449, #6419, #8248 ) ;
#7563=FACE_BOUND ( 'NONE', #8195, .T. ) ;
#7605=EDGE_CURVE ( 'NONE', #18834, #15969, #11470, .T. ) ;
#7606=DIRECTION ( 'NONE',  ( 0.000000000000000000, -1.000000000000000000, 0.000000000000000000 ) ) ;
#7615=ORIENTED_EDGE ( 'NONE', *, *, #14210, .F. ) ;
#7640=AXIS2_PLACEMENT_3D ( 'NONE', #225, #14536, #5388 ) ;
#7682=CARTESIAN_POINT ( 'NONE',  ( -34.99999999999999289, 5.000000000000000000, 9.999999999999971578 ) ) ;
#7692=CIRCLE ( 'NONE', #13526, 59.99999999999703704 ) ;
#7695=AXIS2_PLACEMENT_3D ( 'NONE', #12736, #12956, #16407 ) ;
#7704=CARTESIAN_POINT ( 'NONE',  ( 35.00000000000000000, -5.000000000000000000, 54.99999999999698019 ) ) ;
#7707=VERTEX_POINT ( 'NONE', #21956 ) ;
#7735=AXIS2_PLACEMENT_3D ( 'NONE', #7996, #4786, #4558 ) ;
#7737=ORIENTED_EDGE ( 'NONE', *, *, #7049, .F. ) ;
#7806=UNCERTAINTY_MEASURE_WITH_UNIT (LENGTH_MEASURE( 1.000000000000000082E-05 ), #12569, 'distance_accuracy_value', 'NONE');
#7815=CARTESIAN_POINT ( 'NONE',  ( 89.99999999999701572, -5.000000000000000000, -2.500000000000060840 ) ) ;
#7818=LINE ( 'NONE', #4619, #13422 ) ;
#7855=DIRECTION ( 'NONE',  ( 0.000000000000000000, -1.000000000000000000, 0.000000000000000000 ) ) ;
#7860=LINE ( 'NONE', #6149, #2863 ) ;
#7873=CYLINDRICAL_SURFACE ( 'NONE', #18950, 2.500000000000008882 ) ;
#7877=ADVANCED_FACE ( 'NONE', ( #9086 ), #6626, .T. ) ;
#7902=VECTOR ( 'NONE', #5532, 1000.000000000000000 ) ;
#7931=EDGE_LOOP ( 'NONE', ( #15803, #18692, #16940, #9255 ) ) ;
#7934=FACE_OUTER_BOUND ( 'NONE', #3219, .T. ) ;
#7972=CARTESIAN_POINT ( 'NONE',  ( -34.99999999999999289, 0.000000000000000000, -5.000000000000030198 ) ) ;
#7977=CARTESIAN_POINT ( 'NONE',  ( -34.99999999999999289, -5.000000000000000000, -57.49999999999705125 ) ) ;
#7978=DIRECTION ( 'NONE',  ( 0.000000000000000000, 1.000000000000000000, 0.000000000000000000 ) ) ;
#7981=ADVANCED_FACE ( 'NONE', ( #7934 ), #6100, .F. ) ;
#7996=CARTESIAN_POINT ( 'NONE',  ( -34.99999999999999289, -5.000000000000000000, -3.012171160963566127E-14 ) ) ;
#8013=AXIS2_PLACEMENT_3D ( 'NONE', #5178, #17416, #15355 ) ;
#8014=EDGE_LOOP ( 'NONE', ( #21036, #18314, #12529, #9072 ) ) ;
#8015=VERTEX_POINT ( 'NONE', #22139 ) ;
#8024=DIRECTION ( 'NONE',  ( 0.000000000000000000, 1.000000000000000000, 0.000000000000000000 ) ) ;
#8028=AXIS2_PLACEMENT_3D ( 'NONE', #16705, #15075, #14965 ) ;
#8031=CARTESIAN_POINT ( 'NONE',  ( 35.00000000000001421, 5.000000000000000000, 1.540743955509788682E-30 ) ) ;
#8034=LINE ( 'NONE', #13266, #9995 ) ;
#8060=VECTOR ( 'NONE', #16136, 1000.000000000000000 ) ;
#8064=DIRECTION ( 'NONE',  ( 0.000000000000000000, 0.000000000000000000, 1.000000000000000000 ) ) ;
#8081=EDGE_CURVE ( 'NONE', #13677, #12296, #16127, .T. ) ;
#8096=LINE ( 'NONE', #18389, #1313 ) ;
#8097=DIRECTION ( 'NONE',  ( 8.659560562354903276E-17, -0.7071067811865500152, 0.7071067811865451302 ) ) ;
#8107=ADVANCED_FACE ( 'NONE', ( #1733 ), #20977, .F. ) ;
#8117=ADVANCED_FACE ( 'NONE', ( #3111 ), #4834, .F. ) ;
#8125=ORIENTED_EDGE ( 'NONE', *, *, #2596, .F. ) ;
#8133=DIRECTION ( 'NONE',  ( 0.000000000000000000, 0.000000000000000000, 1.000000000000000000 ) ) ;
#8139=DIRECTION ( 'NONE',  ( 0.000000000000000000, -1.000000000000000000, 0.000000000000000000 ) ) ;
#8159=DIRECTION ( 'NONE',  ( 0.000000000000000000, 0.000000000000000000, -1.000000000000000000 ) ) ;
#8164=CARTESIAN_POINT ( 'NONE',  ( 35.00000000000001421, 0.000000000000000000, 11.00000000000003730 ) ) ;
#8165=DIRECTION ( 'NONE',  ( 0.000000000000000000, -1.000000000000000000, 0.000000000000000000 ) ) ;
#8178=AXIS2_PLACEMENT_3D ( 'NONE', #14362, #18163, #3849 ) ;
#8195=EDGE_LOOP ( 'NONE', ( #8505, #12511 ) ) ;
#8201=AXIS2_PLACEMENT_3D ( 'NONE', #17406, #22360, #1604 ) ;
#8210=MECHANICAL_DESIGN_GEOMETRIC_PRESENTATION_REPRESENTATION('',(#15508),#15874);
#8220=CARTESIAN_POINT ( 'NONE',  ( -0.2854126906104058614, -4.332981472378775401, 48.52899265465749323 ) ) ;
#8221=DIRECTION ( 'NONE',  ( 0.000000000000000000, 0.000000000000000000, 1.000000000000000000 ) ) ;
#8232=EDGE_CURVE ( 'NONE', #12856, #353, #5140, .T. ) ;
#8248=DIRECTION ( 'NONE',  ( 0.000000000000000000, 0.000000000000000000, 1.000000000000000000 ) ) ;
#8294=ORIENTED_EDGE ( 'NONE', *, *, #14501, .F. ) ;
#8297=AXIS2_PLACEMENT_3D ( 'NONE', #8813, #1717, #10289 ) ;
#8304=EDGE_CURVE ( 'NONE', #8525, #16794, #17928, .T. ) ;
#8316=EDGE_LOOP ( 'NONE', ( #3813, #17396 ) ) ;
#8319=ORIENTED_EDGE ( 'NONE', *, *, #7605, .F. ) ;
#8325=CARTESIAN_POINT ( 'NONE',  ( 35.00000000000001421, 1.000000000000044187, 1.540743955509788682E-30 ) ) ;
#8327=EDGE_CURVE ( 'NONE', #11150, #12296, #8934, .T. ) ;
#8390=EDGE_CURVE ( 'NONE', #6061, #9986, #16087, .T. ) ;
#8404=CIRCLE ( 'NONE', #8028, 2.500000000000008882 ) ;
#8424=DIRECTION ( 'NONE',  ( 0.000000000000000000, 1.000000000000000000, 0.000000000000000000 ) ) ;
#8429=ADVANCED_FACE ( 'NONE', ( #4244 ), #9733, .F. ) ;
#8479=EDGE_CURVE ( 'NONE', #14915, #20230, #7692, .T. ) ;
#8480=ADVANCED_FACE ( 'NONE', ( #18326 ), #2643, .T. ) ;
#8487=DIRECTION ( 'NONE',  ( 0.000000000000000000, 0.000000000000000000, 1.000000000000000000 ) ) ;
#8493=EDGE_LOOP ( 'NONE', ( #10447, #9149, #2102, #8294 ) ) ;
#8501=EDGE_CURVE ( 'NONE', #7531, #14915, #20, .T. ) ;
#8505=ORIENTED_EDGE ( 'NONE', *, *, #6388, .T. ) ;
#8515=EDGE_LOOP ( 'NONE', ( #3001, #5105, #11849, #3097 ) ) ;
#8525=VERTEX_POINT ( 'NONE', #9949 ) ;
#8527=DIRECTION ( 'NONE',  ( -0.000000000000000000, -1.000000000000000000, -0.000000000000000000 ) ) ;
#8546=LINE ( 'NONE', #6956, #18623 ) ;
#8561=ADVANCED_FACE ( 'NONE', ( #5156 ), #6408, .F. ) ;
#8571=EDGE_CURVE ( 'NONE', #10113, #2931, #21232, .T. ) ;
#8599=CARTESIAN_POINT ( 'NONE',  ( -34.99999999999999289, 0.000000000000000000, -3.012171160963566127E-14 ) ) ;
#8605=EDGE_CURVE ( 'NONE', #17965, #13528, #13375, .T. ) ;
#8622=ADVANCED_FACE ( 'NONE', ( #20606 ), #5701, .T. ) ;
#8668=CARTESIAN_POINT ( 'NONE',  ( 89.99999999999701572, -5.000000000000000000, -5.216535399428728743E-14 ) ) ;
#8671=FACE_OUTER_BOUND ( 'NONE', #20743, .T. ) ;
#8677=FACE_BOUND ( 'NONE', #982, .T. ) ;
#8711=AXIS2_PLACEMENT_3D ( 'NONE', #12297, #17226, #19301 ) ;
#8719=CARTESIAN_POINT ( 'NONE',  ( 34.99999999999999289, -5.000000000000000000, -54.99999999999705835 ) ) ;
#8756=EDGE_LOOP ( 'NONE', ( #21008, #14176, #1357, #5309 ) ) ;
#8764=VERTEX_POINT ( 'NONE', #22063 ) ;
#8769=VECTOR ( 'NONE', #7040, 1000.000000000000000 ) ;
#8796=FACE_BOUND ( 'NONE', #21451, .T. ) ;
#8813=CARTESIAN_POINT ( 'NONE',  ( -34.99999999999999289, -5.000000000000000000, -3.012171160963566127E-14 ) ) ;
#8842=AXIS2_PLACEMENT_3D ( 'NONE', #17107, #17446, #1424 ) ;
#8880=CARTESIAN_POINT ( 'NONE',  ( 35.00000000000001421, -5.000000000000000000, 59.99999999999703704 ) ) ;
#8886=AXIS2_PLACEMENT_3D ( 'NONE', #19094, #8995, #10591 ) ;
#8895=LINE ( 'NONE', #5244, #21731 ) ;
#8921=AXIS2_PLACEMENT_3D ( 'NONE', #22471, #3563, #10296 ) ;
#8934=LINE ( 'NONE', #17536, #8060 ) ;
#8970=LINE ( 'NONE', #2100, #7902 ) ;
#8995=DIRECTION ( 'NONE',  ( -0.000000000000000000, 1.000000000000000000, -0.000000000000000000 ) ) ;
#8996=CARTESIAN_POINT ( 'NONE',  ( 34.99999999999999289, 0.000000000000000000, -54.99999999999705835 ) ) ;
#9007=CYLINDRICAL_SURFACE ( 'NONE', #13481, 2.500000000000002220 ) ;
#9027=DIRECTION ( 'NONE',  ( 0.000000000000000000, 0.000000000000000000, 1.000000000000000000 ) ) ;
#9038=DIRECTION ( 'NONE',  ( 0.000000000000000000, 0.000000000000000000, 1.000000000000000000 ) ) ;
#9072=ORIENTED_EDGE ( 'NONE', *, *, #15246, .F. ) ;
#9080=VERTEX_POINT ( 'NONE', #2564 ) ;
#9086=FACE_OUTER_BOUND ( 'NONE', #13675, .T. ) ;
#9115=PRODUCT_DEFINITION_FORMATION_WITH_SPECIFIED_SOURCE ( 'ANY', '', #2548, .NOT_KNOWN. ) ;
#9126=DIRECTION ( 'NONE',  ( 0.000000000000000000, 0.000000000000000000, 1.000000000000000000 ) ) ;
#9127=DIRECTION ( 'NONE',  ( 0.000000000000000000, 0.000000000000000000, 1.000000000000000000 ) ) ;
#9131=FACE_BOUND ( 'NONE', #10075, .T. ) ;
#9149=ORIENTED_EDGE ( 'NONE', *, *, #4829, .F. ) ;
#9166=VERTEX_POINT ( 'NONE', #15584 ) ;
#9170=DIRECTION ( 'NONE',  ( 0.000000000000000000, 0.000000000000000000, 1.000000000000000000 ) ) ;
#9190=CARTESIAN_POINT ( 'NONE',  ( -34.99999999999999289, 0.000000000000000000, -3.012171160963566127E-14 ) ) ;
#9255=ORIENTED_EDGE ( 'NONE', *, *, #14210, .T. ) ;
#9340=VERTEX_POINT ( 'NONE', #9406 ) ;
#9358=CARTESIAN_POINT ( 'NONE',  ( 35.00000000000001421, 5.000000000000000000, 1.540743955509788682E-30 ) ) ;
#9404=CARTESIAN_POINT ( 'NONE',  ( 35.00000000000000000, -5.000000000000000000, 54.99999999999698019 ) ) ;
#9406=CARTESIAN_POINT ( 'NONE',  ( 35.00000000000002132, 0.000000000000000000, 58.99999999999702993 ) ) ;
#9424=ORIENTED_EDGE ( 'NONE', *, *, #10161, .F. ) ;
#9458=ORIENTED_EDGE ( 'NONE', *, *, #18151, .T. ) ;
#9468=CIRCLE ( 'NONE', #3976, 10.00000000000000000 ) ;
#9473=PLANE ( 'NONE',  #22310 ) ;
#9475=CONICAL_SURFACE ( 'NONE', #3996, 9.000000000000035527, 0.7853981633974447263 ) ;
#9494=CARTESIAN_POINT ( 'NONE',  ( -34.99999999999998579, -5.000000000000000000, -58.99999999999703704 ) ) ;
#9509=DIRECTION ( 'NONE',  ( 0.000000000000000000, 1.000000000000000000, 0.000000000000000000 ) ) ;
#9510=EDGE_CURVE ( 'NONE', #2931, #10113, #3215, .T. ) ;
#9523=DIRECTION ( 'NONE',  ( 0.000000000000000000, -1.000000000000000000, 0.000000000000000000 ) ) ;
#9525=EDGE_LOOP ( 'NONE', ( #1259, #22319, #6801, #17381 ) ) ;
#9526=EDGE_CURVE ( 'NONE', #5633, #6950, #699, .T. ) ;
#9529=ORIENTED_EDGE ( 'NONE', *, *, #15050, .T. ) ;
#9606=CARTESIAN_POINT ( 'NONE',  ( 35.00000000000000000, 0.000000000000000000, 57.49999999999698730 ) ) ;
#9631=ADVANCED_FACE ( 'NONE', ( #11193 ), #5394, .T. ) ;
#9641=EDGE_LOOP ( 'NONE', ( #3524, #7249, #20475, #21950 ) ) ;
#9658=DIRECTION ( 'NONE',  ( 0.000000000000000000, 1.000000000000000000, 0.000000000000000000 ) ) ;
#9659=EDGE_LOOP ( 'NONE', ( #21951, #10672, #1685, #17825 ) ) ;
#9680=VERTEX_POINT ( 'NONE', #13689 ) ;
#9705=VECTOR ( 'NONE', #2909, 1000.000000000000000 ) ;
#9718=AXIS2_PLACEMENT_3D ( 'NONE', #16561, #7855, #14714 ) ;
#9723=EDGE_CURVE ( 'NONE', #1767, #17965, #21882, .T. ) ;
#9733=PLANE ( 'NONE',  #15723 ) ;
#9791=CARTESIAN_POINT ( 'NONE',  ( 35.00000000000001421, 0.000000000000000000, 1.540743955509788682E-30 ) ) ;
#9795=VECTOR ( 'NONE', #21921, 1000.000000000000114 ) ;
#9824=CIRCLE ( 'NONE', #5804, 2.500000000000008882 ) ;
#9826=DIRECTION ( 'NONE',  ( -0.000000000000000000, 1.000000000000000000, -0.000000000000000000 ) ) ;
#9837=DIRECTION ( 'NONE',  ( 0.000000000000000000, 1.000000000000000000, 0.000000000000000000 ) ) ;
#9839=EDGE_CURVE ( 'NONE', #21906, #9166, #3528, .T. ) ;
#9853=CARTESIAN_POINT ( 'NONE',  ( -34.99999999999999289, 4.000000000000028422, 9.999999999999971578 ) ) ;
#9857=CARTESIAN_POINT ( 'NONE',  ( 35.00000000000001421, 0.000000000000000000, -11.00000000000003730 ) ) ;
#9865=DIRECTION ( 'NONE',  ( 0.000000000000000000, -1.000000000000000000, 0.000000000000000000 ) ) ;
#9876=CARTESIAN_POINT ( 'NONE',  ( -34.99999999999999289, -5.000000000000000000, -57.49999999999705125 ) ) ;
#9887=CYLINDRICAL_SURFACE ( 'NONE', #3631, 59.99999999999703704 ) ;
#9949=CARTESIAN_POINT ( 'NONE',  ( -34.99999999999999289, -5.000000000000000000, -5.000000000000030198 ) ) ;
#9959=CARTESIAN_POINT ( 'NONE',  ( 35.00000000000001421, 0.000000000000000000, 1.540743955509788682E-30 ) ) ;
#9966=EDGE_LOOP ( 'NONE', ( #13352, #2830, #10451, #534 ) ) ;
#9980=CONICAL_SURFACE ( 'NONE', #7416, 59.99999999999700862, 0.7853981633974380649 ) ;
#9982=DIRECTION ( 'NONE',  ( 0.000000000000000000, 0.000000000000000000, 1.000000000000000000 ) ) ;
#9985=CARTESIAN_POINT ( 'NONE',  ( 35.00000000000001421, 5.000000000000000000, -9.000000000000035527 ) ) ;
#9986=VERTEX_POINT ( 'NONE', #13921 ) ;
#9995=VECTOR ( 'NONE', #21669, 1000.000000000000000 ) ;
#10029=CARTESIAN_POINT ( 'NONE',  ( -34.99999999999999289, 1.000000000000044187, 9.999999999999971578 ) ) ;
#10039=VERTEX_POINT ( 'NONE', #19337 ) ;
#10047=EDGE_CURVE ( 'NONE', #8764, #13828, #18217, .T. ) ;
#10060=VECTOR ( 'NONE', #3581, 1000.000000000000000 ) ;
#10075=EDGE_LOOP ( 'NONE', ( #7615, #15556 ) ) ;
#10076=CIRCLE ( 'NONE', #20348, 2.500000000000008882 ) ;
#10098=CIRCLE ( 'NONE', #21085, 59.99999999999703704 ) ;
#10107=EDGE_CURVE ( 'NONE', #17965, #1767, #17118, .T. ) ;
#10113=VERTEX_POINT ( 'NONE', #20234 ) ;
#10117=EDGE_CURVE ( 'NONE', #3077, #9080, #21849, .T. ) ;
#10135=ORIENTED_EDGE ( 'NONE', *, *, #3767, .T. ) ;
#10137=CARTESIAN_POINT ( 'NONE',  ( -34.99999999999997868, -5.000000000000000000, 52.49999999999698730 ) ) ;
#10157=VECTOR ( 'NONE', #4949, 1000.000000000000000 ) ;
#10161=EDGE_CURVE ( 'NONE', #4584, #15969, #5913, .T. ) ;
#10230=DIRECTION ( 'NONE',  ( -0.000000000000000000, -1.000000000000000000, -0.000000000000000000 ) ) ;
#10244=DIRECTION ( 'NONE',  ( 0.000000000000000000, 1.000000000000000000, -0.000000000000000000 ) ) ;
#10264=CARTESIAN_POINT ( 'NONE',  ( -34.99999999999999289, 1.000000000000044187, -10.00000000000003020 ) ) ;
#10282=DIRECTION ( 'NONE',  ( 0.000000000000000000, 0.000000000000000000, 1.000000000000000000 ) ) ;
#10289=DIRECTION ( 'NONE',  ( 0.000000000000000000, 0.000000000000000000, 1.000000000000000000 ) ) ;
#10296=DIRECTION ( 'NONE',  ( 0.000000000000000000, 0.000000000000000000, 1.000000000000000000 ) ) ;
#10298=AXIS2_PLACEMENT_3D ( 'NONE', #16726, #14874, #1035 ) ;
#10311=VERTEX_POINT ( 'NONE', #22526 ) ;
#10337=ORIENTED_EDGE ( 'NONE', *, *, #21970, .T. ) ;
#10340=ORIENTED_EDGE ( 'NONE', *, *, #19895, .F. ) ;
#10341=ORIENTED_EDGE ( 'NONE', *, *, #8081, .F. ) ;
#10342=CARTESIAN_POINT ( 'NONE',  ( -34.99999999999999289, 5.000000000000000000, -3.012171160963566127E-14 ) ) ;
#10347=CARTESIAN_POINT ( 'NONE',  ( 35.00000000000001421, 5.000000000000000000, -9.000000000000035527 ) ) ;
#10350=CARTESIAN_POINT ( 'NONE',  ( -34.99999999999997868, -5.000000000000000000, 57.49999999999699440 ) ) ;
#10372=DIRECTION ( 'NONE',  ( 0.000000000000000000, 0.000000000000000000, 1.000000000000000000 ) ) ;
#10383=ORIENTED_EDGE ( 'NONE', *, *, #18832, .T. ) ;
#10388=DIRECTION ( 'NONE',  ( 0.000000000000000000, 0.000000000000000000, -1.000000000000000000 ) ) ;
#10408=AXIS2_PLACEMENT_3D ( 'NONE', #12115, #5246, #7181 ) ;
#10411=AXIS2_PLACEMENT_3D ( 'NONE', #2392, #4011, #5590 ) ;
#10447=ORIENTED_EDGE ( 'NONE', *, *, #20437, .F. ) ;
#10451=ORIENTED_EDGE ( 'NONE', *, *, #14354, .T. ) ;
#10476=ADVANCED_FACE ( 'NONE', ( #16948 ), #14780, .T. ) ;
#10489=CONICAL_SURFACE ( 'NONE', #624, 9.000000000000035527, 0.7853981633974447263 ) ;
#10506=PRODUCT_DEFINITION ( 'UNKNOWN', '', #9115, #16210 ) ;
#10526=ORIENTED_EDGE ( 'NONE', *, *, #196, .T. ) ;
#10529=ADVANCED_FACE ( 'NONE', ( #15219 ), #6200, .T. ) ;
#10533=DIRECTION ( 'NONE',  ( 0.000000000000000000, 0.000000000000000000, -1.000000000000000000 ) ) ;
#10591=DIRECTION ( 'NONE',  ( 0.000000000000000000, 0.000000000000000000, 1.000000000000000000 ) ) ;
#10605=CARTESIAN_POINT ( 'NONE',  ( 35.00000000000002132, 0.000000000000000000, 58.99999999999701572 ) ) ;
#10615=PLANE ( 'NONE',  #18159 ) ;
#10629=LINE ( 'NONE', #11092, #14019 ) ;
#10638=VERTEX_POINT ( 'NONE', #20966 ) ;
#10639=FACE_BOUND ( 'NONE', #368, .T. ) ;
#10654=MANIFOLD_SOLID_BREP ( 'Chamfer2', #6402 ) ;
#10662=CIRCLE ( 'NONE', #12499, 59.99999999999703704 ) ;
#10672=ORIENTED_EDGE ( 'NONE', *, *, #19848, .F. ) ;
#10682=DIRECTION ( 'NONE',  ( 0.000000000000000000, 0.000000000000000000, 1.000000000000000000 ) ) ;
#10718=EDGE_LOOP ( 'NONE', ( #8319, #1252 ) ) ;
#10735=( NAMED_UNIT ( * ) SI_UNIT ( $, .STERADIAN. ) SOLID_ANGLE_UNIT ( ) );
#10835=FACE_BOUND ( 'NONE', #3244, .T. ) ;
#10844=ADVANCED_FACE ( 'NONE', ( #616 ), #474, .T. ) ;
#10845=EDGE_CURVE ( 'NONE', #15853, #4344, #12580, .T. ) ;
#10853=DIRECTION ( 'NONE',  ( -0.000000000000000000, 1.000000000000000000, -0.000000000000000000 ) ) ;
#10877=FACE_BOUND ( 'NONE', #3148, .T. ) ;
#10896=CIRCLE ( 'NONE', #8711, 59.99999999999700862 ) ;
#10912=VERTEX_POINT ( 'NONE', #16651 ) ;
#10915=AXIS2_PLACEMENT_3D ( 'NONE', #516, #4085, #16446 ) ;
#10919=ORIENTED_EDGE ( 'NONE', *, *, #8501, .T. ) ;
#10988=FACE_OUTER_BOUND ( 'NONE', #19901, .T. ) ;
#10997=FACE_BOUND ( 'NONE', #13730, .T. ) ;
#10999=DIRECTION ( 'NONE',  ( 0.000000000000000000, 0.000000000000000000, -1.000000000000000000 ) ) ;
#11021=DIRECTION ( 'NONE',  ( 0.000000000000000000, -1.000000000000000000, 0.000000000000000000 ) ) ;
#11051=EDGE_CURVE ( 'NONE', #1500, #16627, #8034, .T. ) ;
#11055=VERTEX_POINT ( 'NONE', #14772 ) ;
#11057=CARTESIAN_POINT ( 'NONE',  ( -34.99999999999999289, -5.000000000000000000, -3.012171160963566127E-14 ) ) ;
#11092=CARTESIAN_POINT ( 'NONE',  ( -34.99999999999999289, -5.000000000000000000, -52.49999999999705125 ) ) ;
#11115=CYLINDRICAL_SURFACE ( 'NONE', #21307, 5.000000000000000000 ) ;
#11149=DIRECTION ( 'NONE',  ( 0.000000000000000000, 1.000000000000000000, -0.000000000000000000 ) ) ;
#11150=VERTEX_POINT ( 'NONE', #2990 ) ;
#11153=ADVANCED_FACE ( 'NONE', ( #1490 ), #20275, .T. ) ;
#11157=ORIENTED_EDGE ( 'NONE', *, *, #15425, .F. ) ;
#11172=DIRECTION ( 'NONE',  ( 0.000000000000000000, 0.000000000000000000, 1.000000000000000000 ) ) ;
#11174=VECTOR ( 'NONE', #18534, 1000.000000000000000 ) ;
#11187=DIRECTION ( 'NONE',  ( 0.000000000000000000, 1.000000000000000000, 0.000000000000000000 ) ) ;
#11193=FACE_OUTER_BOUND ( 'NONE', #15583, .T. ) ;
#11201=DIRECTION ( 'NONE',  ( 0.000000000000000000, 0.000000000000000000, 1.000000000000000000 ) ) ;
#11207=DIRECTION ( 'NONE',  ( -0.000000000000000000, -1.000000000000000000, -0.000000000000000000 ) ) ;
#11216=VECTOR ( 'NONE', #20019, 1000.000000000000114 ) ;
#11224=DIRECTION ( 'NONE',  ( -0.000000000000000000, -1.000000000000000000, -0.000000000000000000 ) ) ;
#11225=ORIENTED_EDGE ( 'NONE', *, *, #9723, .T. ) ;
#11237=ORIENTED_EDGE ( 'NONE', *, *, #5832, .F. ) ;
#11245=ORIENTED_EDGE ( 'NONE', *, *, #5518, .T. ) ;
#11261=CONICAL_SURFACE ( 'NONE', #1381, 58.99999999999698730, 0.7853981633974447263 ) ;
#11303=EDGE_LOOP ( 'NONE', ( #6141, #21372, #15426, #830, #6457 ) ) ;
#11309=LINE ( 'NONE', #4211, #7099 ) ;
#11313=DIRECTION ( 'NONE',  ( 0.000000000000000000, -0.7071067811865500152, -0.7071067811865451302 ) ) ;
#11335=EDGE_CURVE ( 'NONE', #19717, #950, #14383, .T. ) ;
#11341=CARTESIAN_POINT ( 'NONE',  ( 35.00000000000001421, 0.000000000000000000, 1.540743955509788682E-30 ) ) ;
#11360=ORIENTED_EDGE ( 'NONE', *, *, #1728, .T. ) ;
#11363=AXIS2_PLACEMENT_3D ( 'NONE', #7704, #18463, #13176 ) ;
#11366=CARTESIAN_POINT ( 'NONE',  ( -2.814138792736986665E-14, -0.3324270965933693867, 47.91030067221368682 ) ) ;
#11390=VERTEX_POINT ( 'NONE', #14637 ) ;
#11391=ORIENTED_EDGE ( 'NONE', *, *, #7511, .F. ) ;
#11400=ORIENTED_EDGE ( 'NONE', *, *, #1264, .T. ) ;
#11407=CARTESIAN_POINT ( 'NONE',  ( -34.99999999999998579, 0.000000000000000000, 58.99999999999695888 ) ) ;
#11408=CIRCLE ( 'NONE', #15416, 58.99999999999699440 ) ;
#11424=CARTESIAN_POINT ( 'NONE',  ( 35.00000000000001421, 5.000000000000000000, 9.000000000000035527 ) ) ;
#11434=DIRECTION ( 'NONE',  ( 0.000000000000000000, 0.000000000000000000, 1.000000000000000000 ) ) ;
#11438=DIRECTION ( 'NONE',  ( 0.000000000000000000, 1.000000000000000000, 0.000000000000000000 ) ) ;
#11455=CARTESIAN_POINT ( 'NONE',  ( -34.99999999999999289, 1.000000000000044187, -10.00000000000003020 ) ) ;
#11459=CARTESIAN_POINT ( 'NONE',  ( 34.99999999999999289, -5.000000000000000000, -54.99999999999705835 ) ) ;
#11464=ADVANCED_FACE ( 'NONE', ( #6175 ), #4458, .T. ) ;
#11469=ORIENTED_EDGE ( 'NONE', *, *, #8327, .T. ) ;
#11470=CIRCLE ( 'NONE', #4539, 2.500000000000002220 ) ;
#11483=LINE ( 'NONE', #16756, #635 ) ;
#11523=CARTESIAN_POINT ( 'NONE',  ( 35.00000000000001421, -1.000000000000028644, 59.99999999999703704 ) ) ;
#11550=VERTEX_POINT ( 'NONE', #10350 ) ;
#11554=DIRECTION ( 'NONE',  ( 0.000000000000000000, 0.000000000000000000, 1.000000000000000000 ) ) ;
#11558=ADVANCED_FACE ( 'NONE', ( #7043 ), #9980, .T. ) ;
#11567=CARTESIAN_POINT ( 'NONE',  ( 35.00000000000001421, -1.000000000000028644, 1.540743955509788682E-30 ) ) ;
#11604=ORIENTED_EDGE ( 'NONE', *, *, #12937, .T. ) ;
#11606=FACE_OUTER_BOUND ( 'NONE', #11303, .T. ) ;
#11612=LINE ( 'NONE', #13876, #18116 ) ;
#11621=CARTESIAN_POINT ( 'NONE',  ( -89.99999999999701572, -5.000000000000000000, -2.500000000000038636 ) ) ;
#11656=CARTESIAN_POINT ( 'NONE',  ( 35.00000000000001421, -5.000000000000000000, 1.540743955509788682E-30 ) ) ;
#11668=DIRECTION ( 'NONE',  ( 0.000000000000000000, 0.000000000000000000, 1.000000000000000000 ) ) ;
#11677=DIRECTION ( 'NONE',  ( -0.000000000000000000, -1.000000000000000000, -0.000000000000000000 ) ) ;
#11723=CARTESIAN_POINT ( 'NONE',  ( 35.00000000000001421, 0.000000000000000000, 1.540743955509788682E-30 ) ) ;
#11762=CARTESIAN_POINT ( 'NONE',  ( -0.8499999999999827693, -5.000000000000000000, 48.11213464397150830 ) ) ;
#11774=CIRCLE ( 'NONE', #10298, 58.99999999999700862 ) ;
#11778=CARTESIAN_POINT ( 'NONE',  ( -89.99999999999701572, -5.000000000000000000, 2.499999999999978684 ) ) ;
#11784=DIRECTION ( 'NONE',  ( 0.000000000000000000, 1.000000000000000000, 0.000000000000000000 ) ) ;
#11832=ORIENTED_EDGE ( 'NONE', *, *, #10845, .T. ) ;
#11836=EDGE_CURVE ( 'NONE', #7707, #4584, #18761, .T. ) ;
#11839=FACE_OUTER_BOUND ( 'NONE', #8493, .T. ) ;
#11849=ORIENTED_EDGE ( 'NONE', *, *, #21699, .T. ) ;
#11863=ORIENTED_EDGE ( 'NONE', *, *, #12254, .F. ) ;
#11883=CARTESIAN_POINT ( 'NONE',  ( -34.99999999999999289, 1.000000000000044187, -3.012171160963566127E-14 ) ) ;
#11900=DIRECTION ( 'NONE',  ( 0.000000000000000000, 0.000000000000000000, 1.000000000000000000 ) ) ;
#11902=DIRECTION ( 'NONE',  ( 0.000000000000000000, 0.000000000000000000, -1.000000000000000000 ) ) ;
#11906=AXIS2_PLACEMENT_3D ( 'NONE', #11656, #664, #4218 ) ;
#12001=VECTOR ( 'NONE', #28, 1000.000000000000000 ) ;
#12047=ORIENTED_EDGE ( 'NONE', *, *, #19895, .T. ) ;
#12067=VECTOR ( 'NONE', #8097, 1000.000000000000114 ) ;
#12089=DIRECTION ( 'NONE',  ( 0.000000000000000000, 1.000000000000000000, -0.000000000000000000 ) ) ;
#12106=DIRECTION ( 'NONE',  ( 0.000000000000000000, 0.000000000000000000, -1.000000000000000000 ) ) ;
#12115=CARTESIAN_POINT ( 'NONE',  ( 35.00000000000001421, 1.000000000000044187, 1.540743955509788682E-30 ) ) ;
#12135=FACE_OUTER_BOUND ( 'NONE', #15475, .T. ) ;
#12143=CARTESIAN_POINT ( 'NONE',  ( 1.387778780781445676E-14, -1.000000000000028644, -48.73397172404115452 ) ) ;
#12175=ORIENTED_EDGE ( 'NONE', *, *, #8501, .F. ) ;
#12196=DIRECTION ( 'NONE',  ( -0.000000000000000000, 1.000000000000000000, -0.000000000000000000 ) ) ;
#12203=ORIENTED_EDGE ( 'NONE', *, *, #1377, .F. ) ;
#12237=DIRECTION ( 'NONE',  ( 0.000000000000000000, 1.000000000000000000, 0.000000000000000000 ) ) ;
#12254=EDGE_CURVE ( 'NONE', #3930, #22344, #15845, .T. ) ;
#12278=DIRECTION ( 'NONE',  ( 0.000000000000000000, 0.000000000000000000, 1.000000000000000000 ) ) ;
#12296=VERTEX_POINT ( 'NONE', #13391 ) ;
#12297=CARTESIAN_POINT ( 'NONE',  ( -34.99999999999999289, -1.000000000000028644, -3.012171160963566127E-14 ) ) ;
#12315=ORIENTED_EDGE ( 'NONE', *, *, #8390, .F. ) ;
#12364=ORIENTED_EDGE ( 'NONE', *, *, #19206, .F. ) ;
#12375=DIRECTION ( 'NONE',  ( 0.000000000000000000, -1.000000000000000000, 0.000000000000000000 ) ) ;
#12384=ORIENTED_EDGE ( 'NONE', *, *, #7133, .F. ) ;
#12393=CIRCLE ( 'NONE', #17516, 4.999999999999997335 ) ;
#12414=EDGE_CURVE ( 'NONE', #11550, #10912, #16855, .T. ) ;
#12448=AXIS2_PLACEMENT_3D ( 'NONE', #2036, #12674, #19695 ) ;
#12450=ADVANCED_FACE ( 'NONE', ( #18913 ), #20745, .F. ) ;
#12482=FACE_OUTER_BOUND ( 'NONE', #22254, .T. ) ;
#12486=CONICAL_SURFACE ( 'NONE', #8842, 9.000000000000035527, 0.7853981633974447263 ) ;
#12499=AXIS2_PLACEMENT_3D ( 'NONE', #13382, #11784, #11900 ) ;
#12511=ORIENTED_EDGE ( 'NONE', *, *, #22531, .T. ) ;
#12523=EDGE_CURVE ( 'NONE', #1500, #11550, #21740, .T. ) ;
#12529=ORIENTED_EDGE ( 'NONE', *, *, #17997, .T. ) ;
#12539=EDGE_LOOP ( 'NONE', ( #18420, #13334, #12175, #3187 ) ) ;
#12546=AXIS2_PLACEMENT_3D ( 'NONE', #19399, #9865, #21792 ) ;
#12548=FACE_OUTER_BOUND ( 'NONE', #2310, .T. ) ;
#12549=AXIS2_PLACEMENT_3D ( 'NONE', #6022, #14605, #2357 ) ;
#12569=( LENGTH_UNIT ( ) NAMED_UNIT ( * ) SI_UNIT ( .MILLI., .METRE. ) );
#12577=EDGE_CURVE ( 'NONE', #10039, #7531, #18762, .T. ) ;
#12580=CIRCLE ( 'NONE', #19156, 2.500000000000002220 ) ;
#12582=CARTESIAN_POINT ( 'NONE',  ( 1.387778780781445676E-14, -3.999999999999985345, -48.73397172404115452 ) ) ;
#12604=EDGE_CURVE ( 'NONE', #2472, #15828, #10629, .T. ) ;
#12625=DIRECTION ( 'NONE',  ( 8.659560562354902043E-17, -0.7071067811865500152, 0.7071067811865450192 ) ) ;
#12674=DIRECTION ( 'NONE',  ( -0.000000000000000000, -1.000000000000000000, -0.000000000000000000 ) ) ;
#12675=DIRECTION ( 'NONE',  ( 0.000000000000000000, -0.000000000000000000, 1.000000000000000000 ) ) ;
#12700=ORIENTED_EDGE ( 'NONE', *, *, #16396, .T. ) ;
#12731=SHAPE_REPRESENTATION_RELATIONSHIP ( 'NONE' , 'NONE' ,  #13507, #4987 ) ;
#12736=CARTESIAN_POINT ( 'NONE',  ( -34.99999999999999289, -5.000000000000000000, -3.012171160963566127E-14 ) ) ;
#12737=CIRCLE ( 'NONE', #18618, 9.000000000000035527 ) ;
#12739=CARTESIAN_POINT ( 'NONE',  ( 35.00000000000001421, 1.000000000000044187, 10.00000000000000000 ) ) ;
#12773=EDGE_LOOP ( 'NONE', ( #20450, #17105, #11863, #13074 ) ) ;
#12818=FACE_BOUND ( 'NONE', #3370, .T. ) ;
#12829=ORIENTED_EDGE ( 'NONE', *, *, #14501, .T. ) ;
#12840=CARTESIAN_POINT ( 'NONE',  ( 35.00000000000000000, -5.000000000000000000, 52.49999999999698019 ) ) ;
#12843=DIRECTION ( 'NONE',  ( 0.000000000000000000, 1.000000000000000000, 0.000000000000000000 ) ) ;
#12854=CARTESIAN_POINT ( 'NONE',  ( 35.00000000000001421, 0.000000000000000000, -4.999999999999997335 ) ) ;
#12856=VERTEX_POINT ( 'NONE', #9606 ) ;
#12858=CYLINDRICAL_SURFACE ( 'NONE', #20846, 2.500000000000002220 ) ;
#12859=DIRECTION ( 'NONE',  ( 0.000000000000000000, 0.000000000000000000, -1.000000000000000000 ) ) ;
#12873=CARTESIAN_POINT ( 'NONE',  ( 1.387778780781445676E-14, -1.000000000000028644, -48.73397172404115452 ) ) ;
#12879=CARTESIAN_POINT ( 'NONE',  ( 34.99999999999999289, -5.000000000000000000, -57.49999999999705835 ) ) ;
#12886=DIRECTION ( 'NONE',  ( 0.000000000000000000, 0.000000000000000000, 1.000000000000000000 ) ) ;
#12892=ORIENTED_EDGE ( 'NONE', *, *, #18740, .T. ) ;
#12929=ORIENTED_EDGE ( 'NONE', *, *, #21865, .T. ) ;
#12937=EDGE_CURVE ( 'NONE', #6950, #4080, #595, .T. ) ;
#12956=DIRECTION ( 'NONE',  ( 0.000000000000000000, 1.000000000000000000, 0.000000000000000000 ) ) ;
#12987=CYLINDRICAL_SURFACE ( 'NONE', #8178, 2.500000000000008882 ) ;
#13002=ORIENTED_EDGE ( 'NONE', *, *, #904, .T. ) ;
#13016=CIRCLE ( 'NONE', #7542, 58.99999999999702283 ) ;
#13049=ORIENTED_EDGE ( 'NONE', *, *, #13220, .F. ) ;
#13069=DIRECTION ( 'NONE',  ( 0.000000000000000000, 0.000000000000000000, 1.000000000000000000 ) ) ;
#13074=ORIENTED_EDGE ( 'NONE', *, *, #17997, .F. ) ;
#13085=AXIS2_PLACEMENT_3D ( 'NONE', #864, #4543, #4429 ) ;
#13087=DIRECTION ( 'NONE',  ( 0.000000000000000000, 0.000000000000000000, -1.000000000000000000 ) ) ;
#13153=DIRECTION ( 'NONE',  ( 0.000000000000000000, 1.000000000000000000, 0.000000000000000000 ) ) ;
#13176=DIRECTION ( 'NONE',  ( 0.000000000000000000, 0.000000000000000000, 1.000000000000000000 ) ) ;
#13177=CYLINDRICAL_SURFACE ( 'NONE', #13896, 2.500000000000002220 ) ;
#13190=ORIENTED_EDGE ( 'NONE', *, *, #15353, .T. ) ;
#13220=EDGE_CURVE ( 'NONE', #7098, #1277, #20242, .T. ) ;
#13224=VERTEX_POINT ( 'NONE', #18395 ) ;
#13246=VECTOR ( 'NONE', #19067, 1000.000000000000114 ) ;
#13257=DIRECTION ( 'NONE',  ( 0.000000000000000000, 0.000000000000000000, 1.000000000000000000 ) ) ;
#13266=CARTESIAN_POINT ( 'NONE',  ( -34.99999999999997868, -5.000000000000000000, 52.49999999999698730 ) ) ;
#13314=DIRECTION ( 'NONE',  ( -0.000000000000000000, -1.000000000000000000, -0.000000000000000000 ) ) ;
#13324=ORIENTED_EDGE ( 'NONE', *, *, #9839, .F. ) ;
#13334=ORIENTED_EDGE ( 'NONE', *, *, #22364, .T. ) ;
#13336=AXIS2_PLACEMENT_3D ( 'NONE', #18829, #1637, #3131 ) ;
#13352=ORIENTED_EDGE ( 'NONE', *, *, #18151, .F. ) ;
#13360=CIRCLE ( 'NONE', #9718, 10.00000000000000000 ) ;
#13362=CARTESIAN_POINT ( 'NONE',  ( -34.99999999999997868, -5.000000000000000000, 54.99999999999698730 ) ) ;
#13375=LINE ( 'NONE', #11778, #17944 ) ;
#13382=CARTESIAN_POINT ( 'NONE',  ( 35.00000000000001421, -5.000000000000000000, 1.540743955509788682E-30 ) ) ;
#13390=CARTESIAN_POINT ( 'NONE',  ( -34.99999999999999289, -5.000000000000000000, 4.999999999999969802 ) ) ;
#13391=CARTESIAN_POINT ( 'NONE',  ( -34.99999999999998579, -1.000000000000028644, -59.99999999999703704 ) ) ;
#13422=VECTOR ( 'NONE', #22031, 1000.000000000000000 ) ;
#13454=VECTOR ( 'NONE', #15462, 1000.000000000000114 ) ;
#13478=DIRECTION ( 'NONE',  ( -0.000000000000000000, 1.000000000000000000, -0.000000000000000000 ) ) ;
#13481=AXIS2_PLACEMENT_3D ( 'NONE', #300, #5915, #9127 ) ;
#13500=ORIENTED_EDGE ( 'NONE', *, *, #2081, .F. ) ;
#13507=SHAPE_REPRESENTATION ( 'FRONT COVER', ( #18273 ), #22681 ) ;
#13522=ORIENTED_EDGE ( 'NONE', *, *, #6770, .T. ) ;
#13526=AXIS2_PLACEMENT_3D ( 'NONE', #4365, #1027, #14868 ) ;
#13528=VERTEX_POINT ( 'NONE', #4063 ) ;
#13529=DIRECTION ( 'NONE',  ( 0.000000000000000000, 0.000000000000000000, -1.000000000000000000 ) ) ;
#13536=DIRECTION ( 'NONE',  ( 0.000000000000000000, 1.000000000000000000, -0.000000000000000000 ) ) ;
#13549=ORIENTED_EDGE ( 'NONE', *, *, #9723, .F. ) ;
#13606=AXIS2_PLACEMENT_3D ( 'NONE', #9791, #13314, #20224 ) ;
#13659=ORIENTED_EDGE ( 'NONE', *, *, #21970, .F. ) ;
#13675=EDGE_LOOP ( 'NONE', ( #1208, #10526, #6938, #20134 ) ) ;
#13677=VERTEX_POINT ( 'NONE', #6671 ) ;
#13689=CARTESIAN_POINT ( 'NONE',  ( 35.00000000000001421, -5.000000000000000000, -4.999999999999997335 ) ) ;
#13700=DIRECTION ( 'NONE',  ( 0.000000000000000000, 0.000000000000000000, 1.000000000000000000 ) ) ;
#13722=CARTESIAN_POINT ( 'NONE',  ( 35.00000000000000000, -5.000000000000000000, 57.49999999999698730 ) ) ;
#13726=CARTESIAN_POINT ( 'NONE',  ( 7.558062341316965381E-15, -0.3324270965933701638, -47.91030067221370103 ) ) ;
#13730=EDGE_LOOP ( 'NONE', ( #16030, #21808 ) ) ;
#13739=DIRECTION ( 'NONE',  ( 0.000000000000000000, 0.000000000000000000, 1.000000000000000000 ) ) ;
#13752=AXIS2_PLACEMENT_3D ( 'NONE', #15128, #2908, #15361 ) ;
#13759=EDGE_CURVE ( 'NONE', #10311, #21906, #6119, .T. ) ;
#13796=AXIS2_PLACEMENT_3D ( 'NONE', #227, #3460, #7218 ) ;
#13803=AXIS2_PLACEMENT_3D ( 'NONE', #6727, #3410, #10372 ) ;
#13805=CARTESIAN_POINT ( 'NONE',  ( -3.469446951953614189E-14, -1.000000000000028644, 48.73397172404114031 ) ) ;
#13821=CIRCLE ( 'NONE', #1757, 2.500000000000002220 ) ;
#13822=DIRECTION ( 'NONE',  ( 0.000000000000000000, -0.000000000000000000, 1.000000000000000000 ) ) ;
#13823=FACE_OUTER_BOUND ( 'NONE', #17901, .T. ) ;
#13828=VERTEX_POINT ( 'NONE', #9494 ) ;
#13830=CONICAL_SURFACE ( 'NONE', #19353, 59.99999999999700862, 0.7853981633974380649 ) ;
#13876=CARTESIAN_POINT ( 'NONE',  ( 89.99999999999701572, -5.000000000000000000, -2.500000000000060840 ) ) ;
#13896=AXIS2_PLACEMENT_3D ( 'NONE', #20194, #12843, #4057 ) ;
#13921=CARTESIAN_POINT ( 'NONE',  ( -0.8499999999999410250, -5.000000000000000000, -48.11213464397154382 ) ) ;
#13957=DIRECTION ( 'NONE',  ( 0.000000000000000000, 0.000000000000000000, 1.000000000000000000 ) ) ;
#13983=CARTESIAN_POINT ( 'NONE',  ( 35.00000000000001421, 1.000000000000044187, 10.00000000000000000 ) ) ;
#13984=CARTESIAN_POINT ( 'NONE',  ( 35.00000000000001421, 0.000000000000000000, 1.540743955509788682E-30 ) ) ;
#14007=ORIENTED_EDGE ( 'NONE', *, *, #1422, .F. ) ;
#14019=VECTOR ( 'NONE', #215, 1000.000000000000000 ) ;
#14045=EDGE_CURVE ( 'NONE', #2875, #4972, #6404, .T. ) ;
#14047=CARTESIAN_POINT ( 'NONE',  ( -89.99999999999701572, -5.000000000000000000, -2.500000000000038636 ) ) ;
#14049=DIRECTION ( 'NONE',  ( 0.000000000000000000, 0.000000000000000000, -1.000000000000000000 ) ) ;
#14100=DIRECTION ( 'NONE',  ( 0.000000000000000000, 0.000000000000000000, 1.000000000000000000 ) ) ;
#14106=EDGE_LOOP ( 'NONE', ( #13659, #18166, #21613, #13049 ) ) ;
#14109=AXIS2_PLACEMENT_3D ( 'NONE', #17652, #5299, #6911 ) ;
#14117=CARTESIAN_POINT ( 'NONE',  ( -34.99999999999999289, 5.000000000000000000, 9.000000000000007105 ) ) ;
#14119=CARTESIAN_POINT ( 'NONE',  ( -89.99999999999701572, -5.000000000000000000, 2.499999999999978684 ) ) ;
#14151=ORIENTED_EDGE ( 'NONE', *, *, #5957, .T. ) ;
#14162=CARTESIAN_POINT ( 'NONE',  ( -34.99999999999999289, 0.000000000000000000, -3.012171160963566127E-14 ) ) ;
#14165=FACE_OUTER_BOUND ( 'NONE', #14106, .T. ) ;
#14166=VECTOR ( 'NONE', #12237, 1000.000000000000000 ) ;
#14176=ORIENTED_EDGE ( 'NONE', *, *, #11051, .T. ) ;
#14190=VERTEX_POINT ( 'NONE', #6179 ) ;
#14192=DIRECTION ( 'NONE',  ( 0.000000000000000000, 1.000000000000000000, -0.000000000000000000 ) ) ;
#14193=ORIENTED_EDGE ( 'NONE', *, *, #10107, .T. ) ;
#14210=EDGE_CURVE ( 'NONE', #15828, #9080, #18475, .T. ) ;
#14211=ORIENTED_EDGE ( 'NONE', *, *, #9526, .F. ) ;
#14216=DIRECTION ( 'NONE',  ( 0.000000000000000000, 0.000000000000000000, 1.000000000000000000 ) ) ;
#14288=ORIENTED_EDGE ( 'NONE', *, *, #22531, .F. ) ;
#14298=ADVANCED_FACE ( 'NONE', ( #6398 ), #20596, .F. ) ;
#14304=CARTESIAN_POINT ( 'NONE',  ( 35.00000000000001421, 0.000000000000000000, -58.99999999999702993 ) ) ;
#14312=CARTESIAN_POINT ( 'NONE',  ( -34.99999999999999289, -5.000000000000000000, -3.012171160963566127E-14 ) ) ;
#14345=ADVANCED_FACE ( 'NONE', ( #13823 ), #20318, .T. ) ;
#14354=EDGE_CURVE ( 'NONE', #9080, #15828, #4935, .T. ) ;
#14362=CARTESIAN_POINT ( 'NONE',  ( 89.99999999999701572, -5.000000000000000000, -5.216535399428728743E-14 ) ) ;
#14376=FACE_OUTER_BOUND ( 'NONE', #7931, .T. ) ;
#14383=CIRCLE ( 'NONE', #3441, 9.000000000000035527 ) ;
#14401=DIRECTION ( 'NONE',  ( 0.000000000000000000, 1.000000000000000000, 0.000000000000000000 ) ) ;
#14426=FACE_OUTER_BOUND ( 'NONE', #15876, .T. ) ;
#14444=AXIS2_PLACEMENT_3D ( 'NONE', #3014, #8165, #9982 ) ;
#14446=CARTESIAN_POINT ( 'NONE',  ( 35.00000000000001421, 0.000000000000000000, 1.540743955509788682E-30 ) ) ;
#14461=DIRECTION ( 'NONE',  ( 0.000000000000000000, 1.000000000000000000, 0.000000000000000000 ) ) ;
#14482=DIRECTION ( 'NONE',  ( 0.000000000000000000, 1.000000000000000000, 0.000000000000000000 ) ) ;
#14501=EDGE_CURVE ( 'NONE', #5633, #2840, #14811, .T. ) ;
#14512=LINE ( 'NONE', #7420, #1778 ) ;
#14527=EDGE_CURVE ( 'NONE', #8525, #4972, #20320, .T. ) ;
#14531=AXIS2_PLACEMENT_3D ( 'NONE', #6776, #20425, #13739 ) ;
#14536=DIRECTION ( 'NONE',  ( 0.000000000000000000, -1.000000000000000000, 0.000000000000000000 ) ) ;
#14548=DIRECTION ( 'NONE',  ( 0.000000000000000000, 0.000000000000000000, 1.000000000000000000 ) ) ;
#14555=VECTOR ( 'NONE', #19169, 1000.000000000000000 ) ;
#14571=DIRECTION ( 'NONE',  ( 0.000000000000000000, -1.000000000000000000, 0.000000000000000000 ) ) ;
#14586=DIRECTION ( 'NONE',  ( 0.000000000000000000, 0.000000000000000000, -1.000000000000000000 ) ) ;
#14605=DIRECTION ( 'NONE',  ( 0.000000000000000000, 1.000000000000000000, 0.000000000000000000 ) ) ;
#14636=FACE_OUTER_BOUND ( 'NONE', #9641, .T. ) ;
#14637=CARTESIAN_POINT ( 'NONE',  ( 35.00000000000001421, 0.000000000000000000, 4.999999999999997335 ) ) ;
#14643=AXIS2_PLACEMENT_3D ( 'NONE', #4809, #11677, #10282 ) ;
#14680=CARTESIAN_POINT ( 'NONE',  ( 35.00000000000001421, 4.000000000000028422, 10.00000000000000000 ) ) ;
#14681=ORIENTED_EDGE ( 'NONE', *, *, #1377, .T. ) ;
#14714=DIRECTION ( 'NONE',  ( 0.000000000000000000, 0.000000000000000000, 1.000000000000000000 ) ) ;
#14741=ORIENTED_EDGE ( 'NONE', *, *, #17581, .T. ) ;
#14761=AXIS2_PLACEMENT_3D ( 'NONE', #1011, #9837, #11434 ) ;
#14772=CARTESIAN_POINT ( 'NONE',  ( -34.99999999999999289, 5.000000000000000000, -9.000000000000065725 ) ) ;
#14780=CONICAL_SURFACE ( 'NONE', #6739, 10.00000000000000000, 0.7853981633974447263 ) ;
#14811=CIRCLE ( 'NONE', #14444, 10.00000000000000000 ) ;
#14836=ORIENTED_EDGE ( 'NONE', *, *, #18832, .F. ) ;
#14868=DIRECTION ( 'NONE',  ( 0.000000000000000000, 0.000000000000000000, 1.000000000000000000 ) ) ;
#14874=DIRECTION ( 'NONE',  ( -0.000000000000000000, -1.000000000000000000, -0.000000000000000000 ) ) ;
#14902=EDGE_CURVE ( 'NONE', #11055, #2840, #20261, .T. ) ;
#14905=ADVANCED_FACE ( 'NONE', ( #6169 ), #4681, .F. ) ;
#14915=VERTEX_POINT ( 'NONE', #16474 ) ;
#14965=DIRECTION ( 'NONE',  ( 0.000000000000000000, 0.000000000000000000, 1.000000000000000000 ) ) ;
#14982=DIRECTION ( 'NONE',  ( 0.000000000000000000, -0.000000000000000000, 1.000000000000000000 ) ) ;
#14990=CARTESIAN_POINT ( 'NONE',  ( 35.00000000000001421, 5.000000000000000000, 1.540743955509788682E-30 ) ) ;
#14991=DIRECTION ( 'NONE',  ( -0.000000000000000000, -1.000000000000000000, -0.000000000000000000 ) ) ;
#14996=APPLICATION_CONTEXT ( 'automotive_design' ) ;
#15003=ORIENTED_EDGE ( 'NONE', *, *, #12523, .T. ) ;
#15013=ORIENTED_EDGE ( 'NONE', *, *, #17180, .F. ) ;
#15032=ADVANCED_FACE ( 'NONE', ( #8671 ), #17368, .F. ) ;
#15050=EDGE_CURVE ( 'NONE', #4972, #2875, #21062, .T. ) ;
#15052=FACE_OUTER_BOUND ( 'NONE', #3815, .T. ) ;
#15075=DIRECTION ( 'NONE',  ( 0.000000000000000000, 1.000000000000000000, 0.000000000000000000 ) ) ;
#15090=DIRECTION ( 'NONE',  ( 0.000000000000000000, -0.000000000000000000, 1.000000000000000000 ) ) ;
#15102=DIRECTION ( 'NONE',  ( 0.000000000000000000, 0.000000000000000000, 1.000000000000000000 ) ) ;
#15128=CARTESIAN_POINT ( 'NONE',  ( -34.99999999999997868, 0.000000000000000000, 54.99999999999698730 ) ) ;
#15219=FACE_OUTER_BOUND ( 'NONE', #7051, .T. ) ;
#15246=EDGE_CURVE ( 'NONE', #22344, #3930, #13360, .T. ) ;
#15250=DIRECTION ( 'NONE',  ( 0.000000000000000000, 1.000000000000000000, -0.000000000000000000 ) ) ;
#15311=ORIENTED_EDGE ( 'NONE', *, *, #3202, .T. ) ;
#15317=AXIS2_PLACEMENT_3D ( 'NONE', #21343, #14571, #21582 ) ;
#15353=EDGE_CURVE ( 'NONE', #9680, #6332, #8096, .T. ) ;
#15355=DIRECTION ( 'NONE',  ( 0.000000000000000000, 0.000000000000000000, -1.000000000000000000 ) ) ;
#15361=DIRECTION ( 'NONE',  ( 0.000000000000000000, 0.000000000000000000, 1.000000000000000000 ) ) ;
#15363=AXIS2_PLACEMENT_3D ( 'NONE', #3907, #3570, #1946 ) ;
#15367=ADVANCED_FACE ( 'NONE', ( #15052 ), #2484, .T. ) ;
#15373=DIRECTION ( 'NONE',  ( 0.000000000000000000, 0.000000000000000000, 1.000000000000000000 ) ) ;
#15393=DIRECTION ( 'NONE',  ( 0.000000000000000000, 0.000000000000000000, 1.000000000000000000 ) ) ;
#15416=AXIS2_PLACEMENT_3D ( 'NONE', #9190, #19409, #3711 ) ;
#15424=ORIENTED_EDGE ( 'NONE', *, *, #15510, .F. ) ;
#15425=EDGE_CURVE ( 'NONE', #10311, #13677, #6595, .T. ) ;
#15426=ORIENTED_EDGE ( 'NONE', *, *, #3932, .T. ) ;
#15442=DIRECTION ( 'NONE',  ( 0.000000000000000000, 1.000000000000000000, 0.000000000000000000 ) ) ;
#15448=CARTESIAN_POINT ( 'NONE',  ( 1.368200027493404197E-14, -0.6657802223429165611, -48.32248901598325119 ) ) ;
#15459=CIRCLE ( 'NONE', #8886, 10.00000000000000000 ) ;
#15462=DIRECTION ( 'NONE',  ( 0.000000000000000000, -0.7071067811865500152, -0.7071067811865451302 ) ) ;
#15475=EDGE_LOOP ( 'NONE', ( #1065, #11469, #19086, #224 ) ) ;
#15483=EDGE_CURVE ( 'NONE', #3496, #10039, #15933, .T. ) ;
#15489=ORIENTED_EDGE ( 'NONE', *, *, #9510, .F. ) ;
#15491=DIRECTION ( 'NONE',  ( 0.000000000000000000, 0.000000000000000000, 1.000000000000000000 ) ) ;
#15498=CARTESIAN_POINT ( 'NONE',  ( -34.99999999999999289, 0.000000000000000000, 4.999999999999969802 ) ) ;
#15508=STYLED_ITEM('',(#22727),#10654);
#15510=EDGE_CURVE ( 'NONE', #5004, #5574, #10076, .T. ) ;
#15556=ORIENTED_EDGE ( 'NONE', *, *, #14354, .F. ) ;
#15583=EDGE_LOOP ( 'NONE', ( #6699, #14836, #11400, #18100 ) ) ;
#15584=CARTESIAN_POINT ( 'NONE',  ( -0.8499999999999827693, -5.000000000000000000, 48.11213464397150830 ) ) ;
#15657=PLANE ( 'NONE',  #1967 ) ;
#15683=EDGE_LOOP ( 'NONE', ( #16588, #19045 ) ) ;
#15691=EDGE_CURVE ( 'NONE', #9986, #2332, #3143, .T. ) ;
#15694=CARTESIAN_POINT ( 'NONE',  ( 89.99999999999701572, -5.000000000000000000, 2.499999999999956479 ) ) ;
#15711=ORIENTED_EDGE ( 'NONE', *, *, #1342, .T. ) ;
#15717=EDGE_CURVE ( 'NONE', #8015, #15814, #21447, .T. ) ;
#15723=AXIS2_PLACEMENT_3D ( 'NONE', #11341, #21656, #15090 ) ;
#15739=CARTESIAN_POINT ( 'NONE',  ( 89.99999999999701572, -5.000000000000000000, -5.216535399428728743E-14 ) ) ;
#15744=AXIS2_PLACEMENT_3D ( 'NONE', #22577, #20852, #1361 ) ;
#15769=EDGE_CURVE ( 'NONE', #9340, #3496, #13016, .T. ) ;
#15771=ORIENTED_EDGE ( 'NONE', *, *, #5547, .F. ) ;
#15775=ORIENTED_EDGE ( 'NONE', *, *, #19535, .T. ) ;
#15803=ORIENTED_EDGE ( 'NONE', *, *, #10117, .F. ) ;
#15814=VERTEX_POINT ( 'NONE', #6643 ) ;
#15828=VERTEX_POINT ( 'NONE', #4715 ) ;
#15845=CIRCLE ( 'NONE', #12546, 10.00000000000000000 ) ;
#15853=VERTEX_POINT ( 'NONE', #13722 ) ;
#15855=DIRECTION ( 'NONE',  ( 0.000000000000000000, 1.000000000000000000, 0.000000000000000000 ) ) ;
#15868=AXIS2_PLACEMENT_3D ( 'NONE', #18360, #15250, #13529 ) ;
#15871=FACE_BOUND ( 'NONE', #5020, .T. ) ;
#15874=( GEOMETRIC_REPRESENTATION_CONTEXT ( 3 ) GLOBAL_UNCERTAINTY_ASSIGNED_CONTEXT ( ( #7806 ) ) GLOBAL_UNIT_ASSIGNED_CONTEXT ( ( #12569, #17627, #10735 ) ) REPRESENTATION_CONTEXT ( 'NONE', 'WORKASPACE' ) );
#15876=EDGE_LOOP ( 'NONE', ( #19578, #8125, #12929, #10341 ) ) ;
#15911=ORIENTED_EDGE ( 'NONE', *, *, #8605, .T. ) ;
#15927=LINE ( 'NONE', #21218, #12001 ) ;
#15933=CIRCLE ( 'NONE', #4606, 58.99999999999702283 ) ;
#15969=VERTEX_POINT ( 'NONE', #672 ) ;
#15977=ADVANCED_FACE ( 'NONE', ( #14636 ), #2393, .T. ) ;
#15982=ORIENTED_EDGE ( 'NONE', *, *, #21865, .F. ) ;
#16030=ORIENTED_EDGE ( 'NONE', *, *, #19848, .T. ) ;
#16042=DIRECTION ( 'NONE',  ( 0.000000000000000000, 0.000000000000000000, -1.000000000000000000 ) ) ;
#16063=CARTESIAN_POINT ( 'NONE',  ( -89.99999999999701572, 0.000000000000000000, -3.012171160963566127E-14 ) ) ;
#16064=DIRECTION ( 'NONE',  ( 0.000000000000000000, 0.000000000000000000, -1.000000000000000000 ) ) ;
#16079=CARTESIAN_POINT ( 'NONE',  ( 35.00000000000001421, 0.000000000000000000, 1.540743955509788682E-30 ) ) ;
#16087=CIRCLE ( 'NONE', #20865, 59.99999999999703704 ) ;
#16098=EDGE_LOOP ( 'NONE', ( #11157, #18726, #10135, #2285 ) ) ;
#16102=DIRECTION ( 'NONE',  ( 0.000000000000000000, -0.000000000000000000, 1.000000000000000000 ) ) ;
#16127=CIRCLE ( 'NONE', #4444, 59.99999999999700862 ) ;
#16136=DIRECTION ( 'NONE',  ( 0.000000000000000000, 1.000000000000000000, 0.000000000000000000 ) ) ;
#16179=ORIENTED_EDGE ( 'NONE', *, *, #7605, .T. ) ;
#16210=PRODUCT_DEFINITION_CONTEXT ( 'detailed design', #14996, 'design' ) ;
#16250=CARTESIAN_POINT ( 'NONE',  ( -34.99999999999999289, 5.000000000000000000, -3.012171160963566127E-14 ) ) ;
#16259=FACE_OUTER_BOUND ( 'NONE', #8014, .T. ) ;
#16281=EDGE_CURVE ( 'NONE', #2472, #3077, #20330, .T. ) ;
#16287=DIRECTION ( 'NONE',  ( 0.000000000000000000, 1.000000000000000000, 0.000000000000000000 ) ) ;
#16291=FACE_OUTER_BOUND ( 'NONE', #8756, .T. ) ;
#16305=VECTOR ( 'NONE', #12625, 1000.000000000000000 ) ;
#16317=EDGE_CURVE ( 'NONE', #22225, #5574, #11612, .T. ) ;
#16329=EDGE_LOOP ( 'NONE', ( #10340, #2234, #21659, #19978 ) ) ;
#16355=CARTESIAN_POINT ( 'NONE',  ( -34.99999999999999289, 1.000000000000044187, -3.012171160963566127E-14 ) ) ;
#16371=CONICAL_SURFACE ( 'NONE', #13796, 58.99999999999698730, 0.7853981633974447263 ) ;
#16396=EDGE_CURVE ( 'NONE', #1277, #17217, #22539, .T. ) ;
#16407=DIRECTION ( 'NONE',  ( 0.000000000000000000, 0.000000000000000000, 1.000000000000000000 ) ) ;
#16413=CIRCLE ( 'NONE', #1791, 10.00000000000000000 ) ;
#16435=CIRCLE ( 'NONE', #15317, 59.99999999999700862 ) ;
#16446=DIRECTION ( 'NONE',  ( 0.000000000000000000, 0.000000000000000000, 1.000000000000000000 ) ) ;
#16448=AXIS2_PLACEMENT_3D ( 'NONE', #4225, #14401, #11201 ) ;
#16455=CARTESIAN_POINT ( 'NONE',  ( -34.99999999999999289, 5.000000000000000000, -3.012171160963566127E-14 ) ) ;
#16474=CARTESIAN_POINT ( 'NONE',  ( 35.00000000000002132, -1.000000000000028644, -59.99999999999703704 ) ) ;
#16485=DIRECTION ( 'NONE',  ( 0.000000000000000000, 0.000000000000000000, 1.000000000000000000 ) ) ;
#16494=ORIENTED_EDGE ( 'NONE', *, *, #12577, .T. ) ;
#16532=EDGE_LOOP ( 'NONE', ( #4311, #6488, #6335, #13 ) ) ;
#16538=CARTESIAN_POINT ( 'NONE',  ( -0.8499999999999410250, -5.000000000000000000, -48.11213464397154382 ) ) ;
#16561=CARTESIAN_POINT ( 'NONE',  ( 35.00000000000001421, 4.000000000000028422, 1.540743955509788682E-30 ) ) ;
#16588=ORIENTED_EDGE ( 'NONE', *, *, #18287, .F. ) ;
#16608=EDGE_CURVE ( 'NONE', #2332, #11150, #21067, .T. ) ;
#16627=VERTEX_POINT ( 'NONE', #7351 ) ;
#16643=AXIS2_PLACEMENT_3D ( 'NONE', #13362, #4689, #11668 ) ;
#16651=CARTESIAN_POINT ( 'NONE',  ( -34.99999999999997868, 0.000000000000000000, 57.49999999999699440 ) ) ;
#16671=AXIS2_PLACEMENT_3D ( 'NONE', #4201, #7978, #11172 ) ;
#16675=DIRECTION ( 'NONE',  ( 0.000000000000000000, 0.000000000000000000, 1.000000000000000000 ) ) ;
#16705=CARTESIAN_POINT ( 'NONE',  ( -89.99999999999701572, 0.000000000000000000, -3.012171160963566127E-14 ) ) ;
#16722=CARTESIAN_POINT ( 'NONE',  ( -34.99999999999997868, -5.000000000000000000, 54.99999999999698730 ) ) ;
#16726=CARTESIAN_POINT ( 'NONE',  ( -34.99999999999999289, -5.000000000000000000, -3.012171160963566127E-14 ) ) ;
#16728=FACE_OUTER_BOUND ( 'NONE', #12773, .T. ) ;
#16747=ORIENTED_EDGE ( 'NONE', *, *, #12254, .T. ) ;
#16756=CARTESIAN_POINT ( 'NONE',  ( -34.99999999999999289, -3.999999999999985345, 59.99999999999698019 ) ) ;
#16764=CARTESIAN_POINT ( 'NONE',  ( 35.00000000000001421, -5.000000000000000000, 1.540743955509788682E-30 ) ) ;
#16765=CIRCLE ( 'NONE', #3963, 9.000000000000035527 ) ;
#16792=CIRCLE ( 'NONE', #8013, 2.500000000000008882 ) ;
#16794=VERTEX_POINT ( 'NONE', #13390 ) ;
#16799=CIRCLE ( 'NONE', #6544, 2.500000000000002220 ) ;
#16802=CARTESIAN_POINT ( 'NONE',  ( -3.469446951953614189E-14, -5.000000000000000000, 48.73397172404114031 ) ) ;
#16811=CYLINDRICAL_SURFACE ( 'NONE', #7735, 59.99999999999700862 ) ;
#16821=PRODUCT_DEFINITION_SHAPE ( 'NONE', 'NONE',  #10506 ) ;
#16822=ORIENTED_EDGE ( 'NONE', *, *, #7049, .T. ) ;
#16846=LINE ( 'NONE', #20063, #17258 ) ;
#16847=EDGE_LOOP ( 'NONE', ( #15982, #13500, #16494, #734 ) ) ;
#16855=LINE ( 'NONE', #19953, #3444 ) ;
#16860=EDGE_LOOP ( 'NONE', ( #5523, #2972, #17502, #6202 ) ) ;
#16868=DIRECTION ( 'NONE',  ( 0.000000000000000000, 1.000000000000000000, -0.000000000000000000 ) ) ;
#16926=EDGE_CURVE ( 'NONE', #10638, #11390, #8970, .T. ) ;
#16940=ORIENTED_EDGE ( 'NONE', *, *, #12604, .T. ) ;
#16948=FACE_OUTER_BOUND ( 'NONE', #21462, .T. ) ;
#16974=CARTESIAN_POINT ( 'NONE',  ( -34.99999999999999289, -5.000000000000000000, -5.000000000000030198 ) ) ;
#16993=DIRECTION ( 'NONE',  ( 1.000000000000000000, 0.000000000000000000, 0.000000000000000000 ) ) ;
#16998=EDGE_LOOP ( 'NONE', ( #717, #1671, #6647, #7494 ) ) ;
#17075=CARTESIAN_POINT ( 'NONE',  ( 34.99999999999999289, -5.000000000000000000, -57.49999999999705835 ) ) ;
#17090=ORIENTED_EDGE ( 'NONE', *, *, #17996, .F. ) ;
#17105=ORIENTED_EDGE ( 'NONE', *, *, #5361, .T. ) ;
#17107=CARTESIAN_POINT ( 'NONE',  ( -34.99999999999999289, 5.000000000000000000, -3.012171160963566127E-14 ) ) ;
#17118=CIRCLE ( 'NONE', #13085, 2.500000000000008882 ) ;
#17120=DIRECTION ( 'NONE',  ( 0.000000000000000000, 1.000000000000000000, 0.000000000000000000 ) ) ;
#17180=EDGE_CURVE ( 'NONE', #10912, #16627, #6089, .T. ) ;
#17217=VERTEX_POINT ( 'NONE', #8164 ) ;
#17226=DIRECTION ( 'NONE',  ( 0.000000000000000000, -1.000000000000000000, 0.000000000000000000 ) ) ;
#17233=DIRECTION ( 'NONE',  ( 0.000000000000000000, 0.000000000000000000, -1.000000000000000000 ) ) ;
#17258=VECTOR ( 'NONE', #18332, 1000.000000000000000 ) ;
#17268=ORIENTED_EDGE ( 'NONE', *, *, #15483, .T. ) ;
#17277=DIRECTION ( 'NONE',  ( 0.000000000000000000, 0.000000000000000000, 1.000000000000000000 ) ) ;
#17293=EDGE_CURVE ( 'NONE', #16794, #2875, #5400, .T. ) ;
#17295=ADVANCED_FACE ( 'NONE', ( #19389 ), #7111, .T. ) ;
#17348=CARTESIAN_POINT ( 'NONE',  ( 35.00000000000001421, 0.000000000000000000, 1.540743955509788682E-30 ) ) ;
#17364=ORIENTED_EDGE ( 'NONE', *, *, #1264, .F. ) ;
#17368=CYLINDRICAL_SURFACE ( 'NONE', #2419, 2.500000000000008882 ) ;
#17372=EDGE_LOOP ( 'NONE', ( #12700, #460 ) ) ;
#17381=ORIENTED_EDGE ( 'NONE', *, *, #22220, .T. ) ;
#17394=DIRECTION ( 'NONE',  ( -0.000000000000000000, -1.000000000000000000, -0.000000000000000000 ) ) ;
#17396=ORIENTED_EDGE ( 'NONE', *, *, #11335, .T. ) ;
#17406=CARTESIAN_POINT ( 'NONE',  ( -34.99999999999997868, -5.000000000000000000, 54.99999999999698730 ) ) ;
#17414=DIRECTION ( 'NONE',  ( 0.000000000000000000, 0.000000000000000000, 1.000000000000000000 ) ) ;
#17416=DIRECTION ( 'NONE',  ( 0.000000000000000000, 1.000000000000000000, -0.000000000000000000 ) ) ;
#17428=EDGE_LOOP ( 'NONE', ( #18271, #12047 ) ) ;
#17446=DIRECTION ( 'NONE',  ( 0.000000000000000000, -1.000000000000000000, 0.000000000000000000 ) ) ;
#17480=DIRECTION ( 'NONE',  ( -0.000000000000000000, -1.000000000000000000, -0.000000000000000000 ) ) ;
#17502=ORIENTED_EDGE ( 'NONE', *, *, #12414, .T. ) ;
#17516=AXIS2_PLACEMENT_3D ( 'NONE', #5393, #2064, #3790 ) ;
#17536=CARTESIAN_POINT ( 'NONE',  ( -34.99999999999998579, -5.000000000000000000, -59.99999999999703704 ) ) ;
#17537=CIRCLE ( 'NONE', #4383, 2.500000000000008882 ) ;
#17541=LINE ( 'NONE', #20641, #10157 ) ;
#17547=ORIENTED_EDGE ( 'NONE', *, *, #3436, .T. ) ;
#17552=ADVANCED_FACE ( 'NONE', ( #14165 ), #18867, .T. ) ;
#17581=EDGE_CURVE ( 'NONE', #13828, #9986, #18118, .T. ) ;
#17605=CARTESIAN_POINT ( 'NONE',  ( 35.00000000000000000, -5.000000000000000000, 54.99999999999698019 ) ) ;
#17624=DIRECTION ( 'NONE',  ( 0.000000000000000000, -1.000000000000000000, 0.000000000000000000 ) ) ;
#17627=( NAMED_UNIT ( * ) PLANE_ANGLE_UNIT ( ) SI_UNIT ( $, .RADIAN. ) );
#17639=DIRECTION ( 'NONE',  ( 0.000000000000000000, 0.000000000000000000, -1.000000000000000000 ) ) ;
#17645=ORIENTED_EDGE ( 'NONE', *, *, #15691, .T. ) ;
#17652=CARTESIAN_POINT ( 'NONE',  ( -34.99999999999999289, -5.000000000000000000, -3.012171160963566127E-14 ) ) ;
#17728=ADVANCED_FACE ( 'NONE', ( #19339 ), #7173, .F. ) ;
#17763=AXIS2_PLACEMENT_3D ( 'NONE', #5932, #10853, #4341 ) ;
#17820=FACE_OUTER_BOUND ( 'NONE', #9659, .T. ) ;
#17825=ORIENTED_EDGE ( 'NONE', *, *, #15510, .T. ) ;
#17830=FACE_OUTER_BOUND ( 'NONE', #17428, .T. ) ;
#17832=DIRECTION ( 'NONE',  ( 8.659560562354903276E-17, -0.7071067811865500152, 0.7071067811865451302 ) ) ;
#17848=ADVANCED_FACE ( 'NONE', ( #14376 ), #9007, .F. ) ;
#17849=DIRECTION ( 'NONE',  ( 0.000000000000000000, -1.000000000000000000, 0.000000000000000000 ) ) ;
#17868=ADVANCED_FACE ( 'NONE', ( #17830 ), #9473, .T. ) ;
#17885=CARTESIAN_POINT ( 'NONE',  ( -34.99999999999999289, -5.000000000000000000, -3.012171160963566127E-14 ) ) ;
#17886=DIRECTION ( 'NONE',  ( 0.000000000000000000, 1.000000000000000000, 0.000000000000000000 ) ) ;
#17901=EDGE_LOOP ( 'NONE', ( #5108, #7737, #21754, #18952 ) ) ;
#17905=DIRECTION ( 'NONE',  ( 0.000000000000000000, 0.000000000000000000, 1.000000000000000000 ) ) ;
#17917=EDGE_CURVE ( 'NONE', #8015, #13677, #1321, .T. ) ;
#17921=ORIENTED_EDGE ( 'NONE', *, *, #9526, .T. ) ;
#17928=CIRCLE ( 'NONE', #15363, 5.000000000000000000 ) ;
#17936=ORIENTED_EDGE ( 'NONE', *, *, #2427, .F. ) ;
#17944=VECTOR ( 'NONE', #18673, 1000.000000000000000 ) ;
#17958=CARTESIAN_POINT ( 'NONE',  ( 35.00000000000000000, -5.000000000000000000, 57.49999999999698730 ) ) ;
#17965=VERTEX_POINT ( 'NONE', #14119 ) ;
#17976=DIRECTION ( 'NONE',  ( -0.000000000000000000, -1.000000000000000000, -0.000000000000000000 ) ) ;
#17982=CARTESIAN_POINT ( 'NONE',  ( 35.00000000000001421, -5.000000000000000000, 1.540743955509788682E-30 ) ) ;
#17996=EDGE_CURVE ( 'NONE', #22225, #2199, #17537, .T. ) ;
#17997=EDGE_CURVE ( 'NONE', #950, #3930, #19081, .T. ) ;
#18011=ORIENTED_EDGE ( 'NONE', *, *, #15353, .F. ) ;
#18030=ADVANCED_FACE ( 'NONE', ( #1039 ), #12858, .F. ) ;
#18032=AXIS2_PLACEMENT_3D ( 'NONE', #22048, #13536, #13087 ) ;
#18047=AXIS2_PLACEMENT_3D ( 'NONE', #16079, #7606, #14586 ) ;
#18098=CARTESIAN_POINT ( 'NONE',  ( 1.387778780781445676E-14, -5.000000000000000000, -1.506085580481783063E-14 ) ) ;
#18100=ORIENTED_EDGE ( 'NONE', *, *, #8571, .F. ) ;
#18116=VECTOR ( 'NONE', #1180, 1000.000000000000000 ) ;
#18118=CIRCLE ( 'NONE', #21413, 58.99999999999700862 ) ;
#18151=EDGE_CURVE ( 'NONE', #3077, #2472, #5474, .T. ) ;
#18159=AXIS2_PLACEMENT_3D ( 'NONE', #14162, #19574, #12675 ) ;
#18163=DIRECTION ( 'NONE',  ( 0.000000000000000000, 1.000000000000000000, 0.000000000000000000 ) ) ;
#18166=ORIENTED_EDGE ( 'NONE', *, *, #1839, .T. ) ;
#18190=DIRECTION ( 'NONE',  ( 0.000000000000000000, -1.000000000000000000, 0.000000000000000000 ) ) ;
#18191=CARTESIAN_POINT ( 'NONE',  ( -34.99999999999999289, 5.000000000000000000, -9.000000000000065725 ) ) ;
#18205=VECTOR ( 'NONE', #4250, 1000.000000000000000 ) ;
#18217=CIRCLE ( 'NONE', #5437, 58.99999999999700862 ) ;
#18224=DIRECTION ( 'NONE',  ( 0.000000000000000000, 0.000000000000000000, 1.000000000000000000 ) ) ;
#18235=AXIS2_PLACEMENT_3D ( 'NONE', #10342, #8527, #1660 ) ;
#18250=DIRECTION ( 'NONE',  ( 0.000000000000000000, 0.000000000000000000, -1.000000000000000000 ) ) ;
#18271=ORIENTED_EDGE ( 'NONE', *, *, #4829, .T. ) ;
#18273=AXIS2_PLACEMENT_3D ( 'NONE', #1648, #15491, #16993 ) ;
#18287=EDGE_CURVE ( 'NONE', #13528, #13224, #8404, .T. ) ;
#18292=CARTESIAN_POINT ( 'NONE',  ( 35.00000000000001421, 1.000000000000044187, -10.00000000000000000 ) ) ;
#18314=ORIENTED_EDGE ( 'NONE', *, *, #19503, .F. ) ;
#18326=FACE_OUTER_BOUND ( 'NONE', #8316, .T. ) ;
#18332=DIRECTION ( 'NONE',  ( 0.000000000000000000, 1.000000000000000000, 0.000000000000000000 ) ) ;
#18352=CARTESIAN_POINT ( 'NONE',  ( -34.99999999999999289, -3.999999999999985345, -3.012171160963566127E-14 ) ) ;
#18360=CARTESIAN_POINT ( 'NONE',  ( 35.00000000000000000, 0.000000000000000000, 54.99999999999698019 ) ) ;
#18371=DIRECTION ( 'NONE',  ( 0.000000000000000000, 1.000000000000000000, 0.000000000000000000 ) ) ;
#18374=AXIS2_PLACEMENT_3D ( 'NONE', #4137, #3916, #16042 ) ;
#18389=CARTESIAN_POINT ( 'NONE',  ( 35.00000000000001421, -5.000000000000000000, -4.999999999999997335 ) ) ;
#18395=CARTESIAN_POINT ( 'NONE',  ( -89.99999999999701572, 0.000000000000000000, -2.500000000000038636 ) ) ;
#18420=ORIENTED_EDGE ( 'NONE', *, *, #15483, .F. ) ;
#18449=CARTESIAN_POINT ( 'NONE',  ( 35.00000000000001421, 0.000000000000000000, 1.540743955509788682E-30 ) ) ;
#18463=DIRECTION ( 'NONE',  ( 0.000000000000000000, 1.000000000000000000, 0.000000000000000000 ) ) ;
#18475=CIRCLE ( 'NONE', #19929, 2.500000000000002220 ) ;
#18506=ORIENTED_EDGE ( 'NONE', *, *, #8327, .F. ) ;
#18534=DIRECTION ( 'NONE',  ( 0.000000000000000000, -0.7071067811865500152, -0.7071067811865450192 ) ) ;
#18554=DIRECTION ( 'NONE',  ( 0.000000000000000000, -1.000000000000000000, 0.000000000000000000 ) ) ;
#18577=ORIENTED_EDGE ( 'NONE', *, *, #16608, .F. ) ;
#18618=AXIS2_PLACEMENT_3D ( 'NONE', #22674, #4789, #3408 ) ;
#18621=ORIENTED_EDGE ( 'NONE', *, *, #16281, .T. ) ;
#18623=VECTOR ( 'NONE', #17480, 1000.000000000000000 ) ;
#18639=ADVANCED_FACE ( 'NONE', ( #16291 ), #13177, .F. ) ;
#18642=ORIENTED_EDGE ( 'NONE', *, *, #19229, .F. ) ;
#18673=DIRECTION ( 'NONE',  ( 0.000000000000000000, 1.000000000000000000, 0.000000000000000000 ) ) ;
#18692=ORIENTED_EDGE ( 'NONE', *, *, #16281, .F. ) ;
#18726=ORIENTED_EDGE ( 'NONE', *, *, #13759, .T. ) ;
#18740=EDGE_CURVE ( 'NONE', #16794, #8525, #4781, .T. ) ;
#18742=CONICAL_SURFACE ( 'NONE', #18374, 58.99999999999698730, 0.7853981633974447263 ) ;
#18761=CIRCLE ( 'NONE', #18032, 2.500000000000002220 ) ;
#18762=B_SPLINE_CURVE_WITH_KNOTS ( 'NONE', 3,
 ( #5169, #13726, #15448, #12143 ),
 .UNSPECIFIED., .F., .F.,
 ( 4, 4 ),
 ( 0.000000000000000000, 0.001590342073036645322 ),
 .UNSPECIFIED. ) ;
#18811=CARTESIAN_POINT ( 'NONE',  ( 35.00000000000001421, 0.000000000000000000, -58.99999999999701572 ) ) ;
#18829=CARTESIAN_POINT ( 'NONE',  ( -34.99999999999999289, -5.000000000000000000, -54.99999999999705125 ) ) ;
#18832=EDGE_CURVE ( 'NONE', #4080, #6950, #5038, .T. ) ;
#18834=VERTEX_POINT ( 'NONE', #20310 ) ;
#18867=CONICAL_SURFACE ( 'NONE', #20331, 10.00000000000000000, 0.7853981633974447263 ) ;
#18913=FACE_OUTER_BOUND ( 'NONE', #21811, .T. ) ;
#18939=ADVANCED_FACE ( 'NONE', ( #5391 ), #11261, .T. ) ;
#18947=CIRCLE ( 'NONE', #4316, 59.99999999999700862 ) ;
#18950=AXIS2_PLACEMENT_3D ( 'NONE', #21862, #6162, #4445 ) ;
#18952=ORIENTED_EDGE ( 'NONE', *, *, #7404, .F. ) ;
#18971=ADVANCED_FACE ( 'NONE', ( #20873 ), #16371, .T. ) ;
#19019=CARTESIAN_POINT ( 'NONE',  ( 35.00000000000001421, 1.000000000000044187, 1.540743955509788682E-30 ) ) ;
#19031=CARTESIAN_POINT ( 'NONE',  ( 35.00000000000001421, 0.000000000000000000, 1.540743955509788682E-30 ) ) ;
#19045=ORIENTED_EDGE ( 'NONE', *, *, #4379, .F. ) ;
#19067=DIRECTION ( 'NONE',  ( 8.659560562354903276E-17, -0.7071067811865500152, 0.7071067811865451302 ) ) ;
#19081=LINE ( 'NONE', #10347, #8769 ) ;
#19086=ORIENTED_EDGE ( 'NONE', *, *, #2868, .T. ) ;
#19094=CARTESIAN_POINT ( 'NONE',  ( 35.00000000000001421, 1.000000000000044187, 1.540743955509788682E-30 ) ) ;
#19106=EDGE_LOOP ( 'NONE', ( #4729, #15003 ) ) ;
#19136=AXIS2_PLACEMENT_3D ( 'NONE', #16722, #6297, #8133 ) ;
#19156=AXIS2_PLACEMENT_3D ( 'NONE', #5890, #11149, #12859 ) ;
#19169=DIRECTION ( 'NONE',  ( -0.000000000000000000, -1.000000000000000000, -0.000000000000000000 ) ) ;
#19206=EDGE_CURVE ( 'NONE', #2199, #5004, #15927, .T. ) ;
#19229=EDGE_CURVE ( 'NONE', #3930, #7098, #2080, .T. ) ;
#19266=DIRECTION ( 'NONE',  ( 0.000000000000000000, 1.000000000000000000, -0.000000000000000000 ) ) ;
#19301=DIRECTION ( 'NONE',  ( 0.000000000000000000, 0.000000000000000000, 1.000000000000000000 ) ) ;
#19334=ORIENTED_EDGE ( 'NONE', *, *, #3932, .F. ) ;
#19337=CARTESIAN_POINT ( 'NONE',  ( 7.943521403985130338E-15, 0.000000000000000000, -47.49736834814795827 ) ) ;
#19339=FACE_OUTER_BOUND ( 'NONE', #16532, .T. ) ;
#19346=VECTOR ( 'NONE', #2710, 1000.000000000000000 ) ;
#19353=AXIS2_PLACEMENT_3D ( 'NONE', #22091, #9826, #9170 ) ;
#19360=CARTESIAN_POINT ( 'NONE',  ( 35.00000000000001421, 4.000000000000028422, -10.00000000000000000 ) ) ;
#19389=FACE_OUTER_BOUND ( 'NONE', #16098, .T. ) ;
#19399=CARTESIAN_POINT ( 'NONE',  ( 35.00000000000001421, 4.000000000000028422, 1.540743955509788682E-30 ) ) ;
#19409=DIRECTION ( 'NONE',  ( 0.000000000000000000, 1.000000000000000000, 0.000000000000000000 ) ) ;
#19411=AXIS2_PLACEMENT_3D ( 'NONE', #19597, #19266, #17639 ) ;
#19433=EDGE_LOOP ( 'NONE', ( #1419, #12203, #13324, #20567 ) ) ;
#19496=CYLINDRICAL_SURFACE ( 'NONE', #14109, 5.000000000000000000 ) ;
#19503=EDGE_CURVE ( 'NONE', #950, #19717, #16765, .T. ) ;
#19535=EDGE_CURVE ( 'NONE', #6950, #10113, #7860, .T. ) ;
#19551=AXIS2_PLACEMENT_3D ( 'NONE', #8031, #14991, #20175 ) ;
#19561=FACE_BOUND ( 'NONE', #10718, .T. ) ;
#19574=DIRECTION ( 'NONE',  ( 0.000000000000000000, 1.000000000000000000, 0.000000000000000000 ) ) ;
#19578=ORIENTED_EDGE ( 'NONE', *, *, #17917, .F. ) ;
#19583=VERTEX_POINT ( 'NONE', #5056 ) ;
#19591=ORIENTED_EDGE ( 'NONE', *, *, #22476, .F. ) ;
#19597=CARTESIAN_POINT ( 'NONE',  ( 35.00000000000000000, 0.000000000000000000, 54.99999999999698019 ) ) ;
#19622=ORIENTED_EDGE ( 'NONE', *, *, #16317, .T. ) ;
#19624=( LENGTH_UNIT ( ) NAMED_UNIT ( * ) SI_UNIT ( .MILLI., .METRE. ) );
#19627=CARTESIAN_POINT ( 'NONE',  ( -3.469446951953614189E-14, -1.000000000000028644, 48.73397172404114031 ) ) ;
#19658=EDGE_CURVE ( 'NONE', #15814, #9340, #20810, .T. ) ;
#19664=DIRECTION ( 'NONE',  ( 0.000000000000000000, 0.000000000000000000, 1.000000000000000000 ) ) ;
#19695=DIRECTION ( 'NONE',  ( 0.000000000000000000, 0.000000000000000000, -1.000000000000000000 ) ) ;
#19717=VERTEX_POINT ( 'NONE', #11424 ) ;
#19718=CONICAL_SURFACE ( 'NONE', #7640, 9.000000000000035527, 0.7853981633974447263 ) ;
#19775=ORIENTED_EDGE ( 'NONE', *, *, #904, .F. ) ;
#19787=DIRECTION ( 'NONE',  ( 0.000000000000000000, 1.000000000000000000, 0.000000000000000000 ) ) ;
#19798=ADVANCED_FACE ( 'NONE', ( #3913 ), #13830, .T. ) ;
#19830=PLANE ( 'NONE',  #4358 ) ;
#19848=EDGE_CURVE ( 'NONE', #2199, #22225, #9824, .T. ) ;
#19889=DIRECTION ( 'NONE',  ( 0.000000000000000000, 1.000000000000000000, 0.000000000000000000 ) ) ;
#19895=EDGE_CURVE ( 'NONE', #19583, #11055, #12737, .T. ) ;
#19901=EDGE_LOOP ( 'NONE', ( #14211, #12829, #14151, #10383 ) ) ;
#19929=AXIS2_PLACEMENT_3D ( 'NONE', #1351, #11438, #11554 ) ;
#19935=CARTESIAN_POINT ( 'NONE',  ( 35.00000000000001421, 5.000000000000000000, 1.540743955509788682E-30 ) ) ;
#19953=CARTESIAN_POINT ( 'NONE',  ( -34.99999999999997868, -5.000000000000000000, 57.49999999999699440 ) ) ;
#19978=ORIENTED_EDGE ( 'NONE', *, *, #14902, .F. ) ;
#20002=AXIS2_PLACEMENT_3D ( 'NONE', #2458, #15442, #15102 ) ;
#20019=DIRECTION ( 'NONE',  ( 0.000000000000000000, -0.7071067811865500152, -0.7071067811865451302 ) ) ;
#20045=AXIS2_PLACEMENT_3D ( 'NONE', #16355, #18190, #20259 ) ;
#20063=CARTESIAN_POINT ( 'NONE',  ( 34.99999999999999289, -5.000000000000000000, -52.49999999999705835 ) ) ;
#20066=CARTESIAN_POINT ( 'NONE',  ( -34.99999999999999289, 1.000000000000044187, -3.012171160963566127E-14 ) ) ;
#20134=ORIENTED_EDGE ( 'NONE', *, *, #22364, .F. ) ;
#20175=DIRECTION ( 'NONE',  ( 0.000000000000000000, 0.000000000000000000, -1.000000000000000000 ) ) ;
#20194=CARTESIAN_POINT ( 'NONE',  ( -34.99999999999997868, -5.000000000000000000, 54.99999999999698730 ) ) ;
#20202=CIRCLE ( 'NONE', #20573, 4.999999999999997335 ) ;
#20211=CARTESIAN_POINT ( 'NONE',  ( -0.5687583343899257349, -4.666323447581314454, -48.32169744526334654 ) ) ;
#20219=ORIENTED_EDGE ( 'NONE', *, *, #15246, .T. ) ;
#20224=DIRECTION ( 'NONE',  ( 0.000000000000000000, 0.000000000000000000, 1.000000000000000000 ) ) ;
#20230=VERTEX_POINT ( 'NONE', #11523 ) ;
#20234=CARTESIAN_POINT ( 'NONE',  ( -34.99999999999999289, 0.000000000000000000, 11.00000000000000888 ) ) ;
#20242=LINE ( 'NONE', #18292, #11216 ) ;
#20259=DIRECTION ( 'NONE',  ( 0.000000000000000000, 0.000000000000000000, -1.000000000000000000 ) ) ;
#20261=LINE ( 'NONE', #18191, #11174 ) ;
#20275=CONICAL_SURFACE ( 'NONE', #1952, 58.99999999999701572, 0.7853981633974447263 ) ;
#20310=CARTESIAN_POINT ( 'NONE',  ( 34.99999999999999289, 0.000000000000000000, -52.49999999999705835 ) ) ;
#20318=CONICAL_SURFACE ( 'NONE', #10408, 10.00000000000000000, 0.7853981633974447263 ) ;
#20320=LINE ( 'NONE', #16974, #9705 ) ;
#20330=CIRCLE ( 'NONE', #13336, 2.500000000000002220 ) ;
#20331=AXIS2_PLACEMENT_3D ( 'NONE', #19019, #17624, #14049 ) ;
#20348=AXIS2_PLACEMENT_3D ( 'NONE', #3280, #10244, #17233 ) ;
#20425=DIRECTION ( 'NONE',  ( -0.000000000000000000, 1.000000000000000000, -0.000000000000000000 ) ) ;
#20437=EDGE_CURVE ( 'NONE', #19583, #5633, #2105, .T. ) ;
#20450=ORIENTED_EDGE ( 'NONE', *, *, #11335, .F. ) ;
#20453=ORIENTED_EDGE ( 'NONE', *, *, #196, .F. ) ;
#20475=ORIENTED_EDGE ( 'NONE', *, *, #5332, .T. ) ;
#20518=AXIS2_PLACEMENT_3D ( 'NONE', #11567, #18554, #2867 ) ;
#20567=ORIENTED_EDGE ( 'NONE', *, *, #13759, .F. ) ;
#20573=AXIS2_PLACEMENT_3D ( 'NONE', #4254, #11224, #18224 ) ;
#20596=CYLINDRICAL_SURFACE ( 'NONE', #16643, 2.500000000000002220 ) ;
#20606=FACE_OUTER_BOUND ( 'NONE', #3758, .T. ) ;
#20641=CARTESIAN_POINT ( 'NONE',  ( 35.00000000000000000, -5.000000000000000000, 52.49999999999698019 ) ) ;
#20653=ORIENTED_EDGE ( 'NONE', *, *, #15050, .F. ) ;
#20670=LINE ( 'NONE', #13983, #13246 ) ;
#20675=CARTESIAN_POINT ( 'NONE',  ( -34.99999999999999289, 4.000000000000028422, -10.00000000000003020 ) ) ;
#20692=ORIENTED_EDGE ( 'NONE', *, *, #19658, .T. ) ;
#20743=EDGE_LOOP ( 'NONE', ( #17090, #19622, #6547, #12364 ) ) ;
#20745=CYLINDRICAL_SURFACE ( 'NONE', #8921, 4.999999999999997335 ) ;
#20808=ADVANCED_FACE ( 'NONE', ( #12482 ), #19496, .F. ) ;
#20810=CIRCLE ( 'NONE', #3982, 58.99999999999702283 ) ;
#20812=CIRCLE ( 'NONE', #10915, 58.99999999999699440 ) ;
#20822=CARTESIAN_POINT ( 'NONE',  ( -3.435937872931129410E-14, -0.6657802223429154509, 48.32248901598323698 ) ) ;
#20825=AXIS2_PLACEMENT_3D ( 'NONE', #17605, #22678, #3530 ) ;
#20846=AXIS2_PLACEMENT_3D ( 'NONE', #11459, #14461, #7271 ) ;
#20848=CARTESIAN_POINT ( 'NONE',  ( 35.00000000000001421, -5.000000000000000000, 59.99999999999703704 ) ) ;
#20852=DIRECTION ( 'NONE',  ( 0.000000000000000000, 1.000000000000000000, 0.000000000000000000 ) ) ;
#20865=AXIS2_PLACEMENT_3D ( 'NONE', #17982, #13153, #2529 ) ;
#20872=CARTESIAN_POINT ( 'NONE',  ( -89.99999999999701572, -5.000000000000000000, -3.012171160963566127E-14 ) ) ;
#20873=FACE_OUTER_BOUND ( 'NONE', #9525, .T. ) ;
#20909=ORIENTED_EDGE ( 'NONE', *, *, #1333, .T. ) ;
#20940=CARTESIAN_POINT ( 'NONE',  ( 89.99999999999701572, -5.000000000000000000, -5.216535399428728743E-14 ) ) ;
#20946=DIRECTION ( 'NONE',  ( 0.000000000000000000, 0.000000000000000000, 1.000000000000000000 ) ) ;
#20966=CARTESIAN_POINT ( 'NONE',  ( 35.00000000000001421, -5.000000000000000000, 4.999999999999997335 ) ) ;
#20977=CYLINDRICAL_SURFACE ( 'NONE', #21601, 2.500000000000008882 ) ;
#21008=ORIENTED_EDGE ( 'NONE', *, *, #12523, .F. ) ;
#21036=ORIENTED_EDGE ( 'NONE', *, *, #5361, .F. ) ;
#21047=DIRECTION ( 'NONE',  ( -0.000000000000000000, -1.000000000000000000, -0.000000000000000000 ) ) ;
#21062=CIRCLE ( 'NONE', #4235, 5.000000000000000000 ) ;
#21067=CIRCLE ( 'NONE', #7157, 59.99999999999700862 ) ;
#21072=ADVANCED_FACE ( 'NONE', ( #16728 ), #10489, .T. ) ;
#21085=AXIS2_PLACEMENT_3D ( 'NONE', #5702, #17849, #9027 ) ;
#21097=FACE_BOUND ( 'NONE', #22055, .T. ) ;
#21163=ADVANCED_FACE ( 'NONE', ( #12135 ), #205, .T. ) ;
#21211=DIRECTION ( 'NONE',  ( 0.000000000000000000, 1.000000000000000000, 0.000000000000000000 ) ) ;
#21218=CARTESIAN_POINT ( 'NONE',  ( 89.99999999999701572, -5.000000000000000000, 2.499999999999956479 ) ) ;
#21232=CIRCLE ( 'NONE', #14643, 11.00000000000003730 ) ;
#21289=CIRCLE ( 'NONE', #5549, 59.99999999999703704 ) ;
#21307=AXIS2_PLACEMENT_3D ( 'NONE', #14312, #17886, #14548 ) ;
#21339=CARTESIAN_POINT ( 'NONE',  ( 35.00000000000001421, -5.000000000000000000, 1.540743955509788682E-30 ) ) ;
#21343=CARTESIAN_POINT ( 'NONE',  ( -34.99999999999999289, -1.000000000000028644, -3.012171160963566127E-14 ) ) ;
#21372=ORIENTED_EDGE ( 'NONE', *, *, #7133, .T. ) ;
#21398=VECTOR ( 'NONE', #181, 1000.000000000000114 ) ;
#21413=AXIS2_PLACEMENT_3D ( 'NONE', #3331, #17394, #17277 ) ;
#21428=FACE_BOUND ( 'NONE', #19106, .T. ) ;
#21447=CIRCLE ( 'NONE', #20002, 58.99999999999699440 ) ;
#21451=EDGE_LOOP ( 'NONE', ( #1360, #19775 ) ) ;
#21462=EDGE_LOOP ( 'NONE', ( #2085, #15775, #15489, #17364 ) ) ;
#21544=DIRECTION ( 'NONE',  ( 0.000000000000000000, 0.000000000000000000, 1.000000000000000000 ) ) ;
#21551=ORIENTED_EDGE ( 'NONE', *, *, #19229, .T. ) ;
#21582=DIRECTION ( 'NONE',  ( -9.251858538543433311E-16, 0.000000000000000000, 1.000000000000000000 ) ) ;
#21601=AXIS2_PLACEMENT_3D ( 'NONE', #20872, #1504, #17414 ) ;
#21602=ORIENTED_EDGE ( 'NONE', *, *, #2596, .T. ) ;
#21607=DIRECTION ( 'NONE',  ( 0.000000000000000000, 1.000000000000000000, -0.000000000000000000 ) ) ;
#21613=ORIENTED_EDGE ( 'NONE', *, *, #16396, .F. ) ;
#21620=CARTESIAN_POINT ( 'NONE',  ( 35.00000000000000000, 0.000000000000000000, 52.49999999999698019 ) ) ;
#21656=DIRECTION ( 'NONE',  ( 0.000000000000000000, 1.000000000000000000, 0.000000000000000000 ) ) ;
#21659=ORIENTED_EDGE ( 'NONE', *, *, #3436, .F. ) ;
#21669=DIRECTION ( 'NONE',  ( 0.000000000000000000, 1.000000000000000000, 0.000000000000000000 ) ) ;
#21699=EDGE_CURVE ( 'NONE', #15969, #18834, #4322, .T. ) ;
#21731=VECTOR ( 'NONE', #6968, 1000.000000000000000 ) ;
#21737=CIRCLE ( 'NONE', #7086, 2.500000000000002220 ) ;
#21740=CIRCLE ( 'NONE', #8201, 2.500000000000002220 ) ;
#21754=ORIENTED_EDGE ( 'NONE', *, *, #13220, .T. ) ;
#21792=DIRECTION ( 'NONE',  ( 0.000000000000000000, 0.000000000000000000, 1.000000000000000000 ) ) ;
#21808=ORIENTED_EDGE ( 'NONE', *, *, #17996, .T. ) ;
#21811=EDGE_LOOP ( 'NONE', ( #14288, #13190, #1345, #5911 ) ) ;
#21819=CARTESIAN_POINT ( 'NONE',  ( 1.387778780781445676E-14, -3.999999999999985345, -48.73397172404115452 ) ) ;
#21849=LINE ( 'NONE', #7977, #19346 ) ;
#21862=CARTESIAN_POINT ( 'NONE',  ( -89.99999999999701572, -5.000000000000000000, -3.012171160963566127E-14 ) ) ;
#21865=EDGE_CURVE ( 'NONE', #14190, #12296, #4333, .T. ) ;
#21882=CIRCLE ( 'NONE', #13803, 2.500000000000008882 ) ;
#21900=ADVANCED_FACE ( 'NONE', ( #4102 ), #7873, .F. ) ;
#21906=VERTEX_POINT ( 'NONE', #5926 ) ;
#21921=DIRECTION ( 'NONE',  ( 8.659560562354844111E-17, 0.7071067811865549002, -0.7071067811865402453 ) ) ;
#21950=ORIENTED_EDGE ( 'NONE', *, *, #5275, .F. ) ;
#21951=ORIENTED_EDGE ( 'NONE', *, *, #16317, .F. ) ;
#21956=CARTESIAN_POINT ( 'NONE',  ( 34.99999999999999289, -5.000000000000000000, -52.49999999999705835 ) ) ;
#21970=EDGE_CURVE ( 'NONE', #3030, #7098, #9468, .T. ) ;
#22007=LINE ( 'NONE', #11455, #74 ) ;
#22031=DIRECTION ( 'NONE',  ( 8.659560562354902043E-17, -0.7071067811865500152, 0.7071067811865450192 ) ) ;
#22032=EDGE_LOOP ( 'NONE', ( #3332, #6516, #17645, #3659, #10919 ) ) ;
#22048=CARTESIAN_POINT ( 'NONE',  ( 34.99999999999999289, -5.000000000000000000, -54.99999999999705835 ) ) ;
#22052=APPLICATION_CONTEXT ( 'automotive_design' ) ;
#22055=EDGE_LOOP ( 'NONE', ( #14193, #11225 ) ) ;
#22063=CARTESIAN_POINT ( 'NONE',  ( -34.99999999999999289, -5.000000000000000000, 58.99999999999698019 ) ) ;
#22091=CARTESIAN_POINT ( 'NONE',  ( -34.99999999999999289, -3.999999999999985345, -3.012171160963566127E-14 ) ) ;
#22101=AXIS2_PLACEMENT_3D ( 'NONE', #13984, #10230, #14100 ) ;
#22139=CARTESIAN_POINT ( 'NONE',  ( -34.99999999999998579, 0.000000000000000000, 58.99999999999697309 ) ) ;
#22167=EDGE_LOOP ( 'NONE', ( #9424, #4887, #20909, #16179 ) ) ;
#22171=ORIENTED_EDGE ( 'NONE', *, *, #2427, .T. ) ;
#22220=EDGE_CURVE ( 'NONE', #4376, #15814, #1452, .T. ) ;
#22225=VERTEX_POINT ( 'NONE', #7815 ) ;
#22248=CIRCLE ( 'NONE', #3206, 2.500000000000008882 ) ;
#22253=AXIS2_PLACEMENT_3D ( 'NONE', #2033, #5700, #10388 ) ;
#22254=EDGE_LOOP ( 'NONE', ( #2782, #993, #3993, #20653 ) ) ;
#22310=AXIS2_PLACEMENT_3D ( 'NONE', #16455, #762, #16102 ) ;
#22319=ORIENTED_EDGE ( 'NONE', *, *, #17917, .T. ) ;
#22344=VERTEX_POINT ( 'NONE', #14680 ) ;
#22360=DIRECTION ( 'NONE',  ( 0.000000000000000000, 1.000000000000000000, 0.000000000000000000 ) ) ;
#22364=EDGE_CURVE ( 'NONE', #3496, #14915, #6557, .T. ) ;
#22385=EDGE_LOOP ( 'NONE', ( #11832, #6407 ) ) ;
#22438=ORIENTED_EDGE ( 'NONE', *, *, #9510, .T. ) ;
#22454=CIRCLE ( 'NONE', #12549, 9.000000000000035527 ) ;
#22467=DIRECTION ( 'NONE',  ( 0.000000000000000000, 0.000000000000000000, -1.000000000000000000 ) ) ;
#22471=CARTESIAN_POINT ( 'NONE',  ( 35.00000000000001421, -5.000000000000000000, 1.540743955509788682E-30 ) ) ;
#22476=EDGE_CURVE ( 'NONE', #5574, #5004, #16792, .T. ) ;
#22526=CARTESIAN_POINT ( 'NONE',  ( -34.99999999999999289, -3.999999999999985345, 59.99999999999698019 ) ) ;
#22531=EDGE_CURVE ( 'NONE', #9680, #10638, #12393, .T. ) ;
#22539=CIRCLE ( 'NONE', #1675, 11.00000000000003730 ) ;
#22562=CARTESIAN_POINT ( 'NONE',  ( 1.387778780781445676E-14, 0.000000000000000000, -1.506085580481783063E-14 ) ) ;
#22577=CARTESIAN_POINT ( 'NONE',  ( -34.99999999999999289, -5.000000000000000000, -54.99999999999705125 ) ) ;
#22674=CARTESIAN_POINT ( 'NONE',  ( -34.99999999999999289, 5.000000000000000000, -3.012171160963566127E-14 ) ) ;
#22678=DIRECTION ( 'NONE',  ( 0.000000000000000000, 1.000000000000000000, 0.000000000000000000 ) ) ;
#22681=( GEOMETRIC_REPRESENTATION_CONTEXT ( 3 ) GLOBAL_UNCERTAINTY_ASSIGNED_CONTEXT ( ( #960 ) ) GLOBAL_UNIT_ASSIGNED_CONTEXT ( ( #19624, #2204, #7472 ) ) REPRESENTATION_CONTEXT ( 'NONE', 'WORKASPACE' ) );
#22684=DIRECTION ( 'NONE',  ( 0.000000000000000000, 1.000000000000000000, 0.000000000000000000 ) ) ;
#22686=ORIENTED_EDGE ( 'NONE', *, *, #17581, .F. ) ;
#22721=COLOUR_RGB('Sky Blue',0.24,0.69,0.87);
#22722=FILL_AREA_STYLE_COLOUR('',#22721);
#22723=FILL_AREA_STYLE('',(#22722));
#22724=SURFACE_STYLE_FILL_AREA(#22723);
#22725=SURFACE_SIDE_STYLE('',(#22724));
#22726=SURFACE_STYLE_USAGE(.BOTH.,#22725);
#22727=PRESENTATION_STYLE_ASSIGNMENT((#22726));
ENDSEC;
END-ISO-10303-21;
